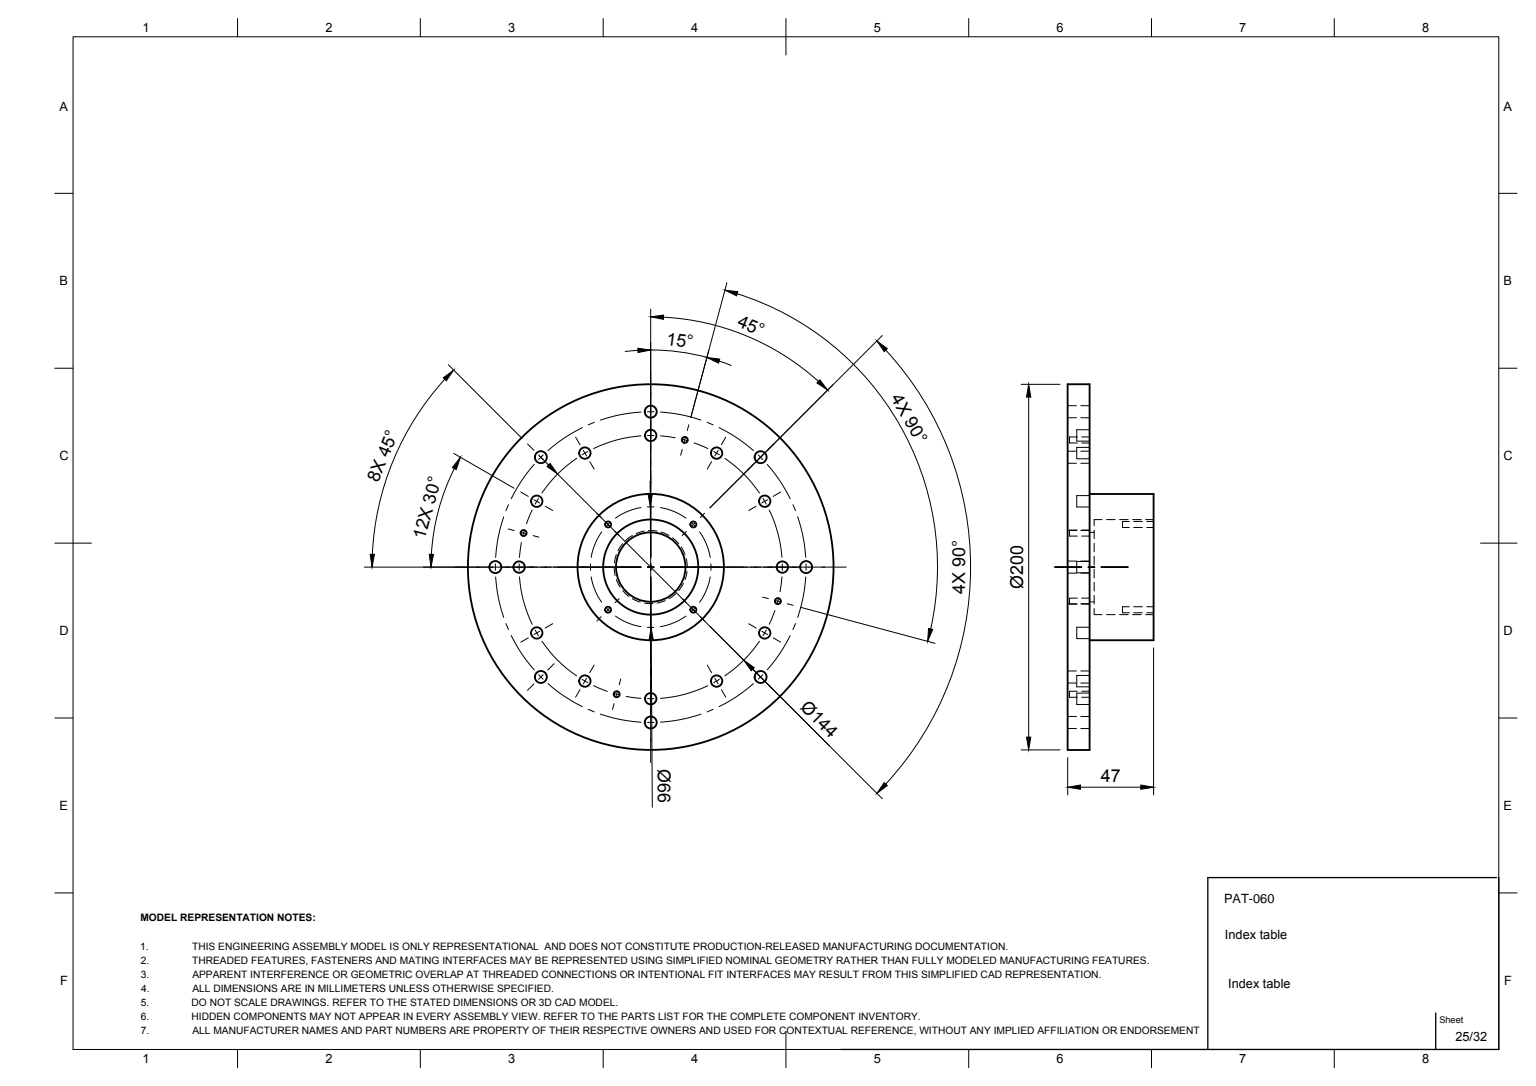
ISO-10303-21;
HEADER;
/* Generated by software containing ST-Developer
 * from STEP Tools, Inc. (www.steptools.com) 
 */

FILE_DESCRIPTION(
/* description */ ('Indexing fixture plate with plunger'),
/* implementation_level */ '2;1');

FILE_NAME(
/* name */ 'Index table.step',
/* time_stamp */ '2026-10-28T03:23:41-07:00',
/* author */ (''),
/* organization */ (''),
/* preprocessor_version */ 'ST-DEVELOPER v20.2',
/* originating_system */ 'Autodesk Translation Framework v15.17.0.0',
/* authorisation */ '');

FILE_SCHEMA (('AUTOMOTIVE_DESIGN { 1 0 10303 214 3 1 1 }'));
ENDSEC;

DATA;
#10=MECHANICAL_DESIGN_GEOMETRIC_PRESENTATION_REPRESENTATION('',(#345),#10020);
#282=SHAPE_REPRESENTATION_RELATIONSHIP('SRR','None',#10158,#309);
#309=ADVANCED_BREP_SHAPE_REPRESENTATION('',(#380),#10011);
#345=STYLED_ITEM('',(#10382),#380);
#380=MANIFOLD_SOLID_BREP('Body1',#4600);
#441=FACE_BOUND('',#1210,.T.);
#442=FACE_BOUND('',#1213,.T.);
#443=FACE_BOUND('',#1215,.T.);
#444=FACE_BOUND('',#1216,.T.);
#445=FACE_BOUND('',#1217,.T.);
#446=FACE_BOUND('',#1218,.T.);
#447=FACE_BOUND('',#1219,.T.);
#448=FACE_BOUND('',#1220,.T.);
#449=FACE_BOUND('',#1221,.T.);
#450=FACE_BOUND('',#1222,.T.);
#451=FACE_BOUND('',#1223,.T.);
#452=FACE_BOUND('',#1224,.T.);
#453=FACE_BOUND('',#1225,.T.);
#454=FACE_BOUND('',#1226,.T.);
#455=FACE_BOUND('',#1227,.T.);
#456=FACE_BOUND('',#1228,.T.);
#457=FACE_BOUND('',#1229,.T.);
#458=FACE_BOUND('',#1230,.T.);
#459=FACE_BOUND('',#1231,.T.);
#460=FACE_BOUND('',#1232,.T.);
#461=FACE_BOUND('',#1233,.T.);
#462=FACE_BOUND('',#1234,.T.);
#463=FACE_BOUND('',#1235,.T.);
#464=FACE_BOUND('',#1236,.T.);
#465=FACE_BOUND('',#1237,.T.);
#466=FACE_BOUND('',#1238,.T.);
#467=FACE_BOUND('',#1239,.T.);
#468=FACE_BOUND('',#1243,.T.);
#469=FACE_BOUND('',#1244,.T.);
#470=FACE_BOUND('',#1245,.T.);
#471=FACE_BOUND('',#1246,.T.);
#472=FACE_BOUND('',#1247,.T.);
#473=FACE_BOUND('',#1248,.T.);
#474=FACE_BOUND('',#1249,.T.);
#475=FACE_BOUND('',#1250,.T.);
#476=FACE_BOUND('',#1251,.T.);
#477=FACE_BOUND('',#1255,.T.);
#478=FACE_BOUND('',#1256,.T.);
#479=FACE_BOUND('',#1257,.T.);
#480=FACE_BOUND('',#1258,.T.);
#481=FACE_BOUND('',#1259,.T.);
#610=PLANE('',#5248);
#611=PLANE('',#5252);
#612=PLANE('',#5256);
#613=PLANE('',#5260);
#614=PLANE('',#5264);
#615=PLANE('',#5268);
#616=PLANE('',#5272);
#617=PLANE('',#5276);
#618=PLANE('',#5280);
#619=PLANE('',#5284);
#620=PLANE('',#5288);
#621=PLANE('',#5292);
#622=PLANE('',#5296);
#623=PLANE('',#5300);
#624=PLANE('',#5304);
#625=PLANE('',#5308);
#626=PLANE('',#5312);
#627=PLANE('',#5316);
#628=PLANE('',#5320);
#629=PLANE('',#5324);
#630=PLANE('',#5349);
#631=PLANE('',#5354);
#632=PLANE('',#5356);
#633=PLANE('',#5363);
#634=PLANE('',#5368);
#821=FACE_OUTER_BOUND('',#1161,.T.);
#822=FACE_OUTER_BOUND('',#1162,.T.);
#823=FACE_OUTER_BOUND('',#1163,.T.);
#824=FACE_OUTER_BOUND('',#1164,.T.);
#825=FACE_OUTER_BOUND('',#1165,.T.);
#826=FACE_OUTER_BOUND('',#1166,.T.);
#827=FACE_OUTER_BOUND('',#1167,.T.);
#828=FACE_OUTER_BOUND('',#1168,.T.);
#829=FACE_OUTER_BOUND('',#1169,.T.);
#830=FACE_OUTER_BOUND('',#1170,.T.);
#831=FACE_OUTER_BOUND('',#1171,.T.);
#832=FACE_OUTER_BOUND('',#1172,.T.);
#833=FACE_OUTER_BOUND('',#1173,.T.);
#834=FACE_OUTER_BOUND('',#1174,.T.);
#835=FACE_OUTER_BOUND('',#1175,.T.);
#836=FACE_OUTER_BOUND('',#1176,.T.);
#837=FACE_OUTER_BOUND('',#1177,.T.);
#838=FACE_OUTER_BOUND('',#1178,.T.);
#839=FACE_OUTER_BOUND('',#1179,.T.);
#840=FACE_OUTER_BOUND('',#1180,.T.);
#841=FACE_OUTER_BOUND('',#1181,.T.);
#842=FACE_OUTER_BOUND('',#1182,.T.);
#843=FACE_OUTER_BOUND('',#1183,.T.);
#844=FACE_OUTER_BOUND('',#1184,.T.);
#845=FACE_OUTER_BOUND('',#1185,.T.);
#846=FACE_OUTER_BOUND('',#1186,.T.);
#847=FACE_OUTER_BOUND('',#1187,.T.);
#848=FACE_OUTER_BOUND('',#1188,.T.);
#849=FACE_OUTER_BOUND('',#1189,.T.);
#850=FACE_OUTER_BOUND('',#1190,.T.);
#851=FACE_OUTER_BOUND('',#1191,.T.);
#852=FACE_OUTER_BOUND('',#1192,.T.);
#853=FACE_OUTER_BOUND('',#1193,.T.);
#854=FACE_OUTER_BOUND('',#1194,.T.);
#855=FACE_OUTER_BOUND('',#1195,.T.);
#856=FACE_OUTER_BOUND('',#1196,.T.);
#857=FACE_OUTER_BOUND('',#1197,.T.);
#858=FACE_OUTER_BOUND('',#1198,.T.);
#859=FACE_OUTER_BOUND('',#1199,.T.);
#860=FACE_OUTER_BOUND('',#1200,.T.);
#861=FACE_OUTER_BOUND('',#1201,.T.);
#862=FACE_OUTER_BOUND('',#1202,.T.);
#863=FACE_OUTER_BOUND('',#1203,.T.);
#864=FACE_OUTER_BOUND('',#1204,.T.);
#865=FACE_OUTER_BOUND('',#1205,.T.);
#866=FACE_OUTER_BOUND('',#1206,.T.);
#867=FACE_OUTER_BOUND('',#1207,.T.);
#868=FACE_OUTER_BOUND('',#1208,.T.);
#869=FACE_OUTER_BOUND('',#1209,.T.);
#870=FACE_OUTER_BOUND('',#1211,.T.);
#871=FACE_OUTER_BOUND('',#1212,.T.);
#872=FACE_OUTER_BOUND('',#1214,.T.);
#873=FACE_OUTER_BOUND('',#1240,.T.);
#874=FACE_OUTER_BOUND('',#1241,.T.);
#875=FACE_OUTER_BOUND('',#1242,.T.);
#876=FACE_OUTER_BOUND('',#1252,.T.);
#877=FACE_OUTER_BOUND('',#1253,.T.);
#878=FACE_OUTER_BOUND('',#1254,.T.);
#1161=EDGE_LOOP('',(#3643,#3644,#3645,#3646));
#1162=EDGE_LOOP('',(#3647));
#1163=EDGE_LOOP('',(#3648,#3649,#3650,#3651));
#1164=EDGE_LOOP('',(#3652));
#1165=EDGE_LOOP('',(#3653,#3654,#3655,#3656));
#1166=EDGE_LOOP('',(#3657));
#1167=EDGE_LOOP('',(#3658,#3659,#3660,#3661));
#1168=EDGE_LOOP('',(#3662));
#1169=EDGE_LOOP('',(#3663,#3664,#3665,#3666));
#1170=EDGE_LOOP('',(#3667));
#1171=EDGE_LOOP('',(#3668,#3669,#3670,#3671));
#1172=EDGE_LOOP('',(#3672));
#1173=EDGE_LOOP('',(#3673,#3674,#3675,#3676));
#1174=EDGE_LOOP('',(#3677));
#1175=EDGE_LOOP('',(#3678,#3679,#3680,#3681));
#1176=EDGE_LOOP('',(#3682));
#1177=EDGE_LOOP('',(#3683,#3684,#3685,#3686));
#1178=EDGE_LOOP('',(#3687));
#1179=EDGE_LOOP('',(#3688,#3689,#3690,#3691));
#1180=EDGE_LOOP('',(#3692));
#1181=EDGE_LOOP('',(#3693,#3694,#3695,#3696));
#1182=EDGE_LOOP('',(#3697));
#1183=EDGE_LOOP('',(#3698,#3699,#3700,#3701));
#1184=EDGE_LOOP('',(#3702));
#1185=EDGE_LOOP('',(#3703,#3704,#3705,#3706));
#1186=EDGE_LOOP('',(#3707));
#1187=EDGE_LOOP('',(#3708,#3709,#3710,#3711));
#1188=EDGE_LOOP('',(#3712));
#1189=EDGE_LOOP('',(#3713,#3714,#3715,#3716));
#1190=EDGE_LOOP('',(#3717));
#1191=EDGE_LOOP('',(#3718,#3719,#3720,#3721));
#1192=EDGE_LOOP('',(#3722));
#1193=EDGE_LOOP('',(#3723,#3724,#3725,#3726));
#1194=EDGE_LOOP('',(#3727));
#1195=EDGE_LOOP('',(#3728,#3729,#3730,#3731));
#1196=EDGE_LOOP('',(#3732));
#1197=EDGE_LOOP('',(#3733,#3734,#3735,#3736));
#1198=EDGE_LOOP('',(#3737));
#1199=EDGE_LOOP('',(#3738,#3739,#3740,#3741));
#1200=EDGE_LOOP('',(#3742));
#1201=EDGE_LOOP('',(#3743,#3744,#3745,#3746));
#1202=EDGE_LOOP('',(#3747,#3748,#3749,#3750));
#1203=EDGE_LOOP('',(#3751,#3752,#3753,#3754));
#1204=EDGE_LOOP('',(#3755,#3756,#3757,#3758));
#1205=EDGE_LOOP('',(#3759,#3760,#3761,#3762));
#1206=EDGE_LOOP('',(#3763,#3764,#3765,#3766));
#1207=EDGE_LOOP('',(#3767,#3768,#3769,#3770));
#1208=EDGE_LOOP('',(#3771,#3772,#3773,#3774));
#1209=EDGE_LOOP('',(#3775));
#1210=EDGE_LOOP('',(#3776));
#1211=EDGE_LOOP('',(#3777,#3778,#3779,#3780));
#1212=EDGE_LOOP('',(#3781));
#1213=EDGE_LOOP('',(#3782));
#1214=EDGE_LOOP('',(#3783));
#1215=EDGE_LOOP('',(#3784));
#1216=EDGE_LOOP('',(#3785));
#1217=EDGE_LOOP('',(#3786));
#1218=EDGE_LOOP('',(#3787));
#1219=EDGE_LOOP('',(#3788));
#1220=EDGE_LOOP('',(#3789));
#1221=EDGE_LOOP('',(#3790));
#1222=EDGE_LOOP('',(#3791));
#1223=EDGE_LOOP('',(#3792));
#1224=EDGE_LOOP('',(#3793));
#1225=EDGE_LOOP('',(#3794));
#1226=EDGE_LOOP('',(#3795));
#1227=EDGE_LOOP('',(#3796));
#1228=EDGE_LOOP('',(#3797));
#1229=EDGE_LOOP('',(#3798));
#1230=EDGE_LOOP('',(#3799));
#1231=EDGE_LOOP('',(#3800));
#1232=EDGE_LOOP('',(#3801));
#1233=EDGE_LOOP('',(#3802));
#1234=EDGE_LOOP('',(#3803));
#1235=EDGE_LOOP('',(#3804));
#1236=EDGE_LOOP('',(#3805));
#1237=EDGE_LOOP('',(#3806));
#1238=EDGE_LOOP('',(#3807));
#1239=EDGE_LOOP('',(#3808));
#1240=EDGE_LOOP('',(#3809,#3810,#3811,#3812));
#1241=EDGE_LOOP('',(#3813,#3814,#3815,#3816));
#1242=EDGE_LOOP('',(#3817));
#1243=EDGE_LOOP('',(#3818));
#1244=EDGE_LOOP('',(#3819));
#1245=EDGE_LOOP('',(#3820));
#1246=EDGE_LOOP('',(#3821));
#1247=EDGE_LOOP('',(#3822));
#1248=EDGE_LOOP('',(#3823));
#1249=EDGE_LOOP('',(#3824));
#1250=EDGE_LOOP('',(#3825));
#1251=EDGE_LOOP('',(#3826));
#1252=EDGE_LOOP('',(#3827,#3828,#3829,#3830));
#1253=EDGE_LOOP('',(#3831,#3832,#3833,#3834));
#1254=EDGE_LOOP('',(#3835));
#1255=EDGE_LOOP('',(#3836));
#1256=EDGE_LOOP('',(#3837));
#1257=EDGE_LOOP('',(#3838));
#1258=EDGE_LOOP('',(#3839));
#1259=EDGE_LOOP('',(#3840));
#1499=LINE('',#9295,#1719);
#1500=LINE('',#9302,#1720);
#1501=LINE('',#9309,#1721);
#1502=LINE('',#9316,#1722);
#1503=LINE('',#9323,#1723);
#1504=LINE('',#9330,#1724);
#1505=LINE('',#9337,#1725);
#1506=LINE('',#9344,#1726);
#1507=LINE('',#9351,#1727);
#1508=LINE('',#9358,#1728);
#1509=LINE('',#9365,#1729);
#1510=LINE('',#9372,#1730);
#1511=LINE('',#9379,#1731);
#1512=LINE('',#9386,#1732);
#1513=LINE('',#9393,#1733);
#1514=LINE('',#9400,#1734);
#1515=LINE('',#9407,#1735);
#1516=LINE('',#9414,#1736);
#1517=LINE('',#9421,#1737);
#1518=LINE('',#9428,#1738);
#1519=LINE('',#9435,#1739);
#1520=LINE('',#9441,#1740);
#1521=LINE('',#9447,#1741);
#1522=LINE('',#9453,#1742);
#1523=LINE('',#9459,#1743);
#1524=LINE('',#9465,#1744);
#1525=LINE('',#9471,#1745);
#1526=LINE('',#9477,#1746);
#1527=LINE('',#9486,#1747);
#1528=LINE('',#9499,#1748);
#1529=LINE('',#9503,#1749);
#1530=LINE('',#9507,#1750);
#1531=LINE('',#9511,#1751);
#1719=VECTOR('',#6360,0.165);
#1720=VECTOR('',#6369,0.165);
#1721=VECTOR('',#6378,0.165);
#1722=VECTOR('',#6387,0.165);
#1723=VECTOR('',#6396,0.31);
#1724=VECTOR('',#6405,0.31);
#1725=VECTOR('',#6414,0.31);
#1726=VECTOR('',#6423,0.31);
#1727=VECTOR('',#6432,0.31);
#1728=VECTOR('',#6441,0.31);
#1729=VECTOR('',#6450,0.31);
#1730=VECTOR('',#6459,0.31);
#1731=VECTOR('',#6468,0.31);
#1732=VECTOR('',#6477,0.31);
#1733=VECTOR('',#6486,0.31);
#1734=VECTOR('',#6495,0.31);
#1735=VECTOR('',#6504,0.165);
#1736=VECTOR('',#6513,0.165);
#1737=VECTOR('',#6522,0.165);
#1738=VECTOR('',#6531,0.165);
#1739=VECTOR('',#6540,0.33);
#1740=VECTOR('',#6547,0.33);
#1741=VECTOR('',#6554,0.33);
#1742=VECTOR('',#6561,0.33);
#1743=VECTOR('',#6568,0.33);
#1744=VECTOR('',#6575,0.33);
#1745=VECTOR('',#6582,0.33);
#1746=VECTOR('',#6589,0.33);
#1747=VECTOR('',#6600,1.9);
#1748=VECTOR('',#6617,2.);
#1749=VECTOR('',#6622,10.);
#1750=VECTOR('',#6627,2.6);
#1751=VECTOR('',#6632,4.);
#1991=CIRCLE('',#5246,0.165);
#1992=CIRCLE('',#5247,0.165);
#1993=CIRCLE('',#5250,0.165);
#1994=CIRCLE('',#5251,0.165);
#1995=CIRCLE('',#5254,0.165);
#1996=CIRCLE('',#5255,0.165);
#1997=CIRCLE('',#5258,0.165);
#1998=CIRCLE('',#5259,0.165);
#1999=CIRCLE('',#5262,0.31);
#2000=CIRCLE('',#5263,0.31);
#2001=CIRCLE('',#5266,0.31);
#2002=CIRCLE('',#5267,0.31);
#2003=CIRCLE('',#5270,0.31);
#2004=CIRCLE('',#5271,0.31);
#2005=CIRCLE('',#5274,0.31);
#2006=CIRCLE('',#5275,0.31);
#2007=CIRCLE('',#5278,0.31);
#2008=CIRCLE('',#5279,0.31);
#2009=CIRCLE('',#5282,0.31);
#2010=CIRCLE('',#5283,0.31);
#2011=CIRCLE('',#5286,0.31);
#2012=CIRCLE('',#5287,0.31);
#2013=CIRCLE('',#5290,0.31);
#2014=CIRCLE('',#5291,0.31);
#2015=CIRCLE('',#5294,0.31);
#2016=CIRCLE('',#5295,0.31);
#2017=CIRCLE('',#5298,0.31);
#2018=CIRCLE('',#5299,0.31);
#2019=CIRCLE('',#5302,0.31);
#2020=CIRCLE('',#5303,0.31);
#2021=CIRCLE('',#5306,0.31);
#2022=CIRCLE('',#5307,0.31);
#2023=CIRCLE('',#5310,0.165);
#2024=CIRCLE('',#5311,0.165);
#2025=CIRCLE('',#5314,0.165);
#2026=CIRCLE('',#5315,0.165);
#2027=CIRCLE('',#5318,0.165);
#2028=CIRCLE('',#5319,0.165);
#2029=CIRCLE('',#5322,0.165);
#2030=CIRCLE('',#5323,0.165);
#2031=CIRCLE('',#5326,0.33);
#2032=CIRCLE('',#5327,0.33);
#2033=CIRCLE('',#5329,0.33);
#2034=CIRCLE('',#5330,0.33);
#2035=CIRCLE('',#5332,0.33);
#2036=CIRCLE('',#5333,0.33);
#2037=CIRCLE('',#5335,0.33);
#2038=CIRCLE('',#5336,0.33);
#2039=CIRCLE('',#5338,0.33);
#2040=CIRCLE('',#5339,0.33);
#2041=CIRCLE('',#5341,0.33);
#2042=CIRCLE('',#5342,0.33);
#2043=CIRCLE('',#5344,0.33);
#2044=CIRCLE('',#5345,0.33);
#2045=CIRCLE('',#5347,0.33);
#2046=CIRCLE('',#5348,0.33);
#2047=CIRCLE('',#5350,2.);
#2048=CIRCLE('',#5351,1.9);
#2049=CIRCLE('',#5353,1.9);
#2050=CIRCLE('',#5355,2.6);
#2051=CIRCLE('',#5357,10.);
#2052=CIRCLE('',#5358,4.);
#2053=CIRCLE('',#5360,2.);
#2054=CIRCLE('',#5362,10.);
#2055=CIRCLE('',#5365,2.6);
#2056=CIRCLE('',#5367,4.);
#2338=VERTEX_POINT('',#9292);
#2339=VERTEX_POINT('',#9294);
#2340=VERTEX_POINT('',#9299);
#2341=VERTEX_POINT('',#9301);
#2342=VERTEX_POINT('',#9306);
#2343=VERTEX_POINT('',#9308);
#2344=VERTEX_POINT('',#9313);
#2345=VERTEX_POINT('',#9315);
#2346=VERTEX_POINT('',#9320);
#2347=VERTEX_POINT('',#9322);
#2348=VERTEX_POINT('',#9327);
#2349=VERTEX_POINT('',#9329);
#2350=VERTEX_POINT('',#9334);
#2351=VERTEX_POINT('',#9336);
#2352=VERTEX_POINT('',#9341);
#2353=VERTEX_POINT('',#9343);
#2354=VERTEX_POINT('',#9348);
#2355=VERTEX_POINT('',#9350);
#2356=VERTEX_POINT('',#9355);
#2357=VERTEX_POINT('',#9357);
#2358=VERTEX_POINT('',#9362);
#2359=VERTEX_POINT('',#9364);
#2360=VERTEX_POINT('',#9369);
#2361=VERTEX_POINT('',#9371);
#2362=VERTEX_POINT('',#9376);
#2363=VERTEX_POINT('',#9378);
#2364=VERTEX_POINT('',#9383);
#2365=VERTEX_POINT('',#9385);
#2366=VERTEX_POINT('',#9390);
#2367=VERTEX_POINT('',#9392);
#2368=VERTEX_POINT('',#9397);
#2369=VERTEX_POINT('',#9399);
#2370=VERTEX_POINT('',#9404);
#2371=VERTEX_POINT('',#9406);
#2372=VERTEX_POINT('',#9411);
#2373=VERTEX_POINT('',#9413);
#2374=VERTEX_POINT('',#9418);
#2375=VERTEX_POINT('',#9420);
#2376=VERTEX_POINT('',#9425);
#2377=VERTEX_POINT('',#9427);
#2378=VERTEX_POINT('',#9432);
#2379=VERTEX_POINT('',#9434);
#2380=VERTEX_POINT('',#9438);
#2381=VERTEX_POINT('',#9440);
#2382=VERTEX_POINT('',#9444);
#2383=VERTEX_POINT('',#9446);
#2384=VERTEX_POINT('',#9450);
#2385=VERTEX_POINT('',#9452);
#2386=VERTEX_POINT('',#9456);
#2387=VERTEX_POINT('',#9458);
#2388=VERTEX_POINT('',#9462);
#2389=VERTEX_POINT('',#9464);
#2390=VERTEX_POINT('',#9468);
#2391=VERTEX_POINT('',#9470);
#2392=VERTEX_POINT('',#9474);
#2393=VERTEX_POINT('',#9476);
#2394=VERTEX_POINT('',#9480);
#2395=VERTEX_POINT('',#9482);
#2396=VERTEX_POINT('',#9485);
#2397=VERTEX_POINT('',#9489);
#2398=VERTEX_POINT('',#9492);
#2399=VERTEX_POINT('',#9494);
#2400=VERTEX_POINT('',#9497);
#2401=VERTEX_POINT('',#9501);
#2402=VERTEX_POINT('',#9506);
#2403=VERTEX_POINT('',#9510);
#2801=EDGE_CURVE('',#2338,#2338,#1991,.T.);
#2802=EDGE_CURVE('',#2338,#2339,#1499,.T.);
#2803=EDGE_CURVE('',#2339,#2339,#1992,.T.);
#2804=EDGE_CURVE('',#2340,#2340,#1993,.T.);
#2805=EDGE_CURVE('',#2340,#2341,#1500,.T.);
#2806=EDGE_CURVE('',#2341,#2341,#1994,.T.);
#2807=EDGE_CURVE('',#2342,#2342,#1995,.T.);
#2808=EDGE_CURVE('',#2342,#2343,#1501,.T.);
#2809=EDGE_CURVE('',#2343,#2343,#1996,.T.);
#2810=EDGE_CURVE('',#2344,#2344,#1997,.T.);
#2811=EDGE_CURVE('',#2344,#2345,#1502,.T.);
#2812=EDGE_CURVE('',#2345,#2345,#1998,.T.);
#2813=EDGE_CURVE('',#2346,#2346,#1999,.T.);
#2814=EDGE_CURVE('',#2346,#2347,#1503,.T.);
#2815=EDGE_CURVE('',#2347,#2347,#2000,.T.);
#2816=EDGE_CURVE('',#2348,#2348,#2001,.T.);
#2817=EDGE_CURVE('',#2348,#2349,#1504,.T.);
#2818=EDGE_CURVE('',#2349,#2349,#2002,.T.);
#2819=EDGE_CURVE('',#2350,#2350,#2003,.T.);
#2820=EDGE_CURVE('',#2350,#2351,#1505,.T.);
#2821=EDGE_CURVE('',#2351,#2351,#2004,.T.);
#2822=EDGE_CURVE('',#2352,#2352,#2005,.T.);
#2823=EDGE_CURVE('',#2352,#2353,#1506,.T.);
#2824=EDGE_CURVE('',#2353,#2353,#2006,.T.);
#2825=EDGE_CURVE('',#2354,#2354,#2007,.T.);
#2826=EDGE_CURVE('',#2354,#2355,#1507,.T.);
#2827=EDGE_CURVE('',#2355,#2355,#2008,.T.);
#2828=EDGE_CURVE('',#2356,#2356,#2009,.T.);
#2829=EDGE_CURVE('',#2356,#2357,#1508,.T.);
#2830=EDGE_CURVE('',#2357,#2357,#2010,.T.);
#2831=EDGE_CURVE('',#2358,#2358,#2011,.T.);
#2832=EDGE_CURVE('',#2358,#2359,#1509,.T.);
#2833=EDGE_CURVE('',#2359,#2359,#2012,.T.);
#2834=EDGE_CURVE('',#2360,#2360,#2013,.T.);
#2835=EDGE_CURVE('',#2360,#2361,#1510,.T.);
#2836=EDGE_CURVE('',#2361,#2361,#2014,.T.);
#2837=EDGE_CURVE('',#2362,#2362,#2015,.T.);
#2838=EDGE_CURVE('',#2362,#2363,#1511,.T.);
#2839=EDGE_CURVE('',#2363,#2363,#2016,.T.);
#2840=EDGE_CURVE('',#2364,#2364,#2017,.T.);
#2841=EDGE_CURVE('',#2364,#2365,#1512,.T.);
#2842=EDGE_CURVE('',#2365,#2365,#2018,.T.);
#2843=EDGE_CURVE('',#2366,#2366,#2019,.T.);
#2844=EDGE_CURVE('',#2366,#2367,#1513,.T.);
#2845=EDGE_CURVE('',#2367,#2367,#2020,.T.);
#2846=EDGE_CURVE('',#2368,#2368,#2021,.T.);
#2847=EDGE_CURVE('',#2368,#2369,#1514,.T.);
#2848=EDGE_CURVE('',#2369,#2369,#2022,.T.);
#2849=EDGE_CURVE('',#2370,#2370,#2023,.T.);
#2850=EDGE_CURVE('',#2370,#2371,#1515,.T.);
#2851=EDGE_CURVE('',#2371,#2371,#2024,.T.);
#2852=EDGE_CURVE('',#2372,#2372,#2025,.T.);
#2853=EDGE_CURVE('',#2372,#2373,#1516,.T.);
#2854=EDGE_CURVE('',#2373,#2373,#2026,.T.);
#2855=EDGE_CURVE('',#2374,#2374,#2027,.T.);
#2856=EDGE_CURVE('',#2374,#2375,#1517,.T.);
#2857=EDGE_CURVE('',#2375,#2375,#2028,.T.);
#2858=EDGE_CURVE('',#2376,#2376,#2029,.T.);
#2859=EDGE_CURVE('',#2376,#2377,#1518,.T.);
#2860=EDGE_CURVE('',#2377,#2377,#2030,.T.);
#2861=EDGE_CURVE('',#2378,#2378,#2031,.T.);
#2862=EDGE_CURVE('',#2378,#2379,#1519,.T.);
#2863=EDGE_CURVE('',#2379,#2379,#2032,.T.);
#2864=EDGE_CURVE('',#2380,#2380,#2033,.T.);
#2865=EDGE_CURVE('',#2380,#2381,#1520,.T.);
#2866=EDGE_CURVE('',#2381,#2381,#2034,.T.);
#2867=EDGE_CURVE('',#2382,#2382,#2035,.T.);
#2868=EDGE_CURVE('',#2382,#2383,#1521,.T.);
#2869=EDGE_CURVE('',#2383,#2383,#2036,.T.);
#2870=EDGE_CURVE('',#2384,#2384,#2037,.T.);
#2871=EDGE_CURVE('',#2384,#2385,#1522,.T.);
#2872=EDGE_CURVE('',#2385,#2385,#2038,.T.);
#2873=EDGE_CURVE('',#2386,#2386,#2039,.T.);
#2874=EDGE_CURVE('',#2386,#2387,#1523,.T.);
#2875=EDGE_CURVE('',#2387,#2387,#2040,.T.);
#2876=EDGE_CURVE('',#2388,#2388,#2041,.T.);
#2877=EDGE_CURVE('',#2388,#2389,#1524,.T.);
#2878=EDGE_CURVE('',#2389,#2389,#2042,.T.);
#2879=EDGE_CURVE('',#2390,#2390,#2043,.T.);
#2880=EDGE_CURVE('',#2390,#2391,#1525,.T.);
#2881=EDGE_CURVE('',#2391,#2391,#2044,.T.);
#2882=EDGE_CURVE('',#2392,#2392,#2045,.T.);
#2883=EDGE_CURVE('',#2392,#2393,#1526,.T.);
#2884=EDGE_CURVE('',#2393,#2393,#2046,.T.);
#2885=EDGE_CURVE('',#2394,#2394,#2047,.T.);
#2886=EDGE_CURVE('',#2395,#2395,#2048,.T.);
#2887=EDGE_CURVE('',#2395,#2396,#1527,.T.);
#2888=EDGE_CURVE('',#2396,#2396,#2049,.T.);
#2889=EDGE_CURVE('',#2397,#2397,#2050,.T.);
#2890=EDGE_CURVE('',#2398,#2398,#2051,.T.);
#2891=EDGE_CURVE('',#2399,#2399,#2052,.T.);
#2892=EDGE_CURVE('',#2400,#2400,#2053,.T.);
#2893=EDGE_CURVE('',#2400,#2394,#1528,.T.);
#2894=EDGE_CURVE('',#2401,#2401,#2054,.T.);
#2895=EDGE_CURVE('',#2401,#2398,#1529,.T.);
#2896=EDGE_CURVE('',#2397,#2402,#1530,.T.);
#2897=EDGE_CURVE('',#2402,#2402,#2055,.T.);
#2898=EDGE_CURVE('',#2399,#2403,#1531,.T.);
#2899=EDGE_CURVE('',#2403,#2403,#2056,.T.);
#3643=ORIENTED_EDGE('',*,*,#2801,.F.);
#3644=ORIENTED_EDGE('',*,*,#2802,.T.);
#3645=ORIENTED_EDGE('',*,*,#2803,.T.);
#3646=ORIENTED_EDGE('',*,*,#2802,.F.);
#3647=ORIENTED_EDGE('',*,*,#2803,.F.);
#3648=ORIENTED_EDGE('',*,*,#2804,.F.);
#3649=ORIENTED_EDGE('',*,*,#2805,.T.);
#3650=ORIENTED_EDGE('',*,*,#2806,.T.);
#3651=ORIENTED_EDGE('',*,*,#2805,.F.);
#3652=ORIENTED_EDGE('',*,*,#2806,.F.);
#3653=ORIENTED_EDGE('',*,*,#2807,.F.);
#3654=ORIENTED_EDGE('',*,*,#2808,.T.);
#3655=ORIENTED_EDGE('',*,*,#2809,.T.);
#3656=ORIENTED_EDGE('',*,*,#2808,.F.);
#3657=ORIENTED_EDGE('',*,*,#2809,.F.);
#3658=ORIENTED_EDGE('',*,*,#2810,.F.);
#3659=ORIENTED_EDGE('',*,*,#2811,.T.);
#3660=ORIENTED_EDGE('',*,*,#2812,.T.);
#3661=ORIENTED_EDGE('',*,*,#2811,.F.);
#3662=ORIENTED_EDGE('',*,*,#2812,.F.);
#3663=ORIENTED_EDGE('',*,*,#2813,.F.);
#3664=ORIENTED_EDGE('',*,*,#2814,.T.);
#3665=ORIENTED_EDGE('',*,*,#2815,.T.);
#3666=ORIENTED_EDGE('',*,*,#2814,.F.);
#3667=ORIENTED_EDGE('',*,*,#2815,.F.);
#3668=ORIENTED_EDGE('',*,*,#2816,.F.);
#3669=ORIENTED_EDGE('',*,*,#2817,.T.);
#3670=ORIENTED_EDGE('',*,*,#2818,.T.);
#3671=ORIENTED_EDGE('',*,*,#2817,.F.);
#3672=ORIENTED_EDGE('',*,*,#2818,.F.);
#3673=ORIENTED_EDGE('',*,*,#2819,.F.);
#3674=ORIENTED_EDGE('',*,*,#2820,.T.);
#3675=ORIENTED_EDGE('',*,*,#2821,.T.);
#3676=ORIENTED_EDGE('',*,*,#2820,.F.);
#3677=ORIENTED_EDGE('',*,*,#2821,.F.);
#3678=ORIENTED_EDGE('',*,*,#2822,.F.);
#3679=ORIENTED_EDGE('',*,*,#2823,.T.);
#3680=ORIENTED_EDGE('',*,*,#2824,.T.);
#3681=ORIENTED_EDGE('',*,*,#2823,.F.);
#3682=ORIENTED_EDGE('',*,*,#2824,.F.);
#3683=ORIENTED_EDGE('',*,*,#2825,.F.);
#3684=ORIENTED_EDGE('',*,*,#2826,.T.);
#3685=ORIENTED_EDGE('',*,*,#2827,.T.);
#3686=ORIENTED_EDGE('',*,*,#2826,.F.);
#3687=ORIENTED_EDGE('',*,*,#2827,.F.);
#3688=ORIENTED_EDGE('',*,*,#2828,.F.);
#3689=ORIENTED_EDGE('',*,*,#2829,.T.);
#3690=ORIENTED_EDGE('',*,*,#2830,.T.);
#3691=ORIENTED_EDGE('',*,*,#2829,.F.);
#3692=ORIENTED_EDGE('',*,*,#2830,.F.);
#3693=ORIENTED_EDGE('',*,*,#2831,.F.);
#3694=ORIENTED_EDGE('',*,*,#2832,.T.);
#3695=ORIENTED_EDGE('',*,*,#2833,.T.);
#3696=ORIENTED_EDGE('',*,*,#2832,.F.);
#3697=ORIENTED_EDGE('',*,*,#2833,.F.);
#3698=ORIENTED_EDGE('',*,*,#2834,.F.);
#3699=ORIENTED_EDGE('',*,*,#2835,.T.);
#3700=ORIENTED_EDGE('',*,*,#2836,.T.);
#3701=ORIENTED_EDGE('',*,*,#2835,.F.);
#3702=ORIENTED_EDGE('',*,*,#2836,.F.);
#3703=ORIENTED_EDGE('',*,*,#2837,.F.);
#3704=ORIENTED_EDGE('',*,*,#2838,.T.);
#3705=ORIENTED_EDGE('',*,*,#2839,.T.);
#3706=ORIENTED_EDGE('',*,*,#2838,.F.);
#3707=ORIENTED_EDGE('',*,*,#2839,.F.);
#3708=ORIENTED_EDGE('',*,*,#2840,.F.);
#3709=ORIENTED_EDGE('',*,*,#2841,.T.);
#3710=ORIENTED_EDGE('',*,*,#2842,.T.);
#3711=ORIENTED_EDGE('',*,*,#2841,.F.);
#3712=ORIENTED_EDGE('',*,*,#2842,.F.);
#3713=ORIENTED_EDGE('',*,*,#2843,.F.);
#3714=ORIENTED_EDGE('',*,*,#2844,.T.);
#3715=ORIENTED_EDGE('',*,*,#2845,.T.);
#3716=ORIENTED_EDGE('',*,*,#2844,.F.);
#3717=ORIENTED_EDGE('',*,*,#2845,.F.);
#3718=ORIENTED_EDGE('',*,*,#2846,.F.);
#3719=ORIENTED_EDGE('',*,*,#2847,.T.);
#3720=ORIENTED_EDGE('',*,*,#2848,.T.);
#3721=ORIENTED_EDGE('',*,*,#2847,.F.);
#3722=ORIENTED_EDGE('',*,*,#2848,.F.);
#3723=ORIENTED_EDGE('',*,*,#2849,.F.);
#3724=ORIENTED_EDGE('',*,*,#2850,.T.);
#3725=ORIENTED_EDGE('',*,*,#2851,.T.);
#3726=ORIENTED_EDGE('',*,*,#2850,.F.);
#3727=ORIENTED_EDGE('',*,*,#2851,.F.);
#3728=ORIENTED_EDGE('',*,*,#2852,.F.);
#3729=ORIENTED_EDGE('',*,*,#2853,.T.);
#3730=ORIENTED_EDGE('',*,*,#2854,.T.);
#3731=ORIENTED_EDGE('',*,*,#2853,.F.);
#3732=ORIENTED_EDGE('',*,*,#2854,.F.);
#3733=ORIENTED_EDGE('',*,*,#2855,.F.);
#3734=ORIENTED_EDGE('',*,*,#2856,.T.);
#3735=ORIENTED_EDGE('',*,*,#2857,.T.);
#3736=ORIENTED_EDGE('',*,*,#2856,.F.);
#3737=ORIENTED_EDGE('',*,*,#2857,.F.);
#3738=ORIENTED_EDGE('',*,*,#2858,.F.);
#3739=ORIENTED_EDGE('',*,*,#2859,.T.);
#3740=ORIENTED_EDGE('',*,*,#2860,.T.);
#3741=ORIENTED_EDGE('',*,*,#2859,.F.);
#3742=ORIENTED_EDGE('',*,*,#2860,.F.);
#3743=ORIENTED_EDGE('',*,*,#2861,.F.);
#3744=ORIENTED_EDGE('',*,*,#2862,.T.);
#3745=ORIENTED_EDGE('',*,*,#2863,.F.);
#3746=ORIENTED_EDGE('',*,*,#2862,.F.);
#3747=ORIENTED_EDGE('',*,*,#2864,.F.);
#3748=ORIENTED_EDGE('',*,*,#2865,.T.);
#3749=ORIENTED_EDGE('',*,*,#2866,.F.);
#3750=ORIENTED_EDGE('',*,*,#2865,.F.);
#3751=ORIENTED_EDGE('',*,*,#2867,.F.);
#3752=ORIENTED_EDGE('',*,*,#2868,.T.);
#3753=ORIENTED_EDGE('',*,*,#2869,.F.);
#3754=ORIENTED_EDGE('',*,*,#2868,.F.);
#3755=ORIENTED_EDGE('',*,*,#2870,.F.);
#3756=ORIENTED_EDGE('',*,*,#2871,.T.);
#3757=ORIENTED_EDGE('',*,*,#2872,.F.);
#3758=ORIENTED_EDGE('',*,*,#2871,.F.);
#3759=ORIENTED_EDGE('',*,*,#2873,.F.);
#3760=ORIENTED_EDGE('',*,*,#2874,.T.);
#3761=ORIENTED_EDGE('',*,*,#2875,.F.);
#3762=ORIENTED_EDGE('',*,*,#2874,.F.);
#3763=ORIENTED_EDGE('',*,*,#2876,.F.);
#3764=ORIENTED_EDGE('',*,*,#2877,.T.);
#3765=ORIENTED_EDGE('',*,*,#2878,.F.);
#3766=ORIENTED_EDGE('',*,*,#2877,.F.);
#3767=ORIENTED_EDGE('',*,*,#2879,.F.);
#3768=ORIENTED_EDGE('',*,*,#2880,.T.);
#3769=ORIENTED_EDGE('',*,*,#2881,.F.);
#3770=ORIENTED_EDGE('',*,*,#2880,.F.);
#3771=ORIENTED_EDGE('',*,*,#2882,.F.);
#3772=ORIENTED_EDGE('',*,*,#2883,.T.);
#3773=ORIENTED_EDGE('',*,*,#2884,.F.);
#3774=ORIENTED_EDGE('',*,*,#2883,.F.);
#3775=ORIENTED_EDGE('',*,*,#2885,.F.);
#3776=ORIENTED_EDGE('',*,*,#2886,.T.);
#3777=ORIENTED_EDGE('',*,*,#2886,.F.);
#3778=ORIENTED_EDGE('',*,*,#2887,.T.);
#3779=ORIENTED_EDGE('',*,*,#2888,.T.);
#3780=ORIENTED_EDGE('',*,*,#2887,.F.);
#3781=ORIENTED_EDGE('',*,*,#2889,.F.);
#3782=ORIENTED_EDGE('',*,*,#2888,.F.);
#3783=ORIENTED_EDGE('',*,*,#2890,.F.);
#3784=ORIENTED_EDGE('',*,*,#2813,.T.);
#3785=ORIENTED_EDGE('',*,*,#2816,.T.);
#3786=ORIENTED_EDGE('',*,*,#2819,.T.);
#3787=ORIENTED_EDGE('',*,*,#2822,.T.);
#3788=ORIENTED_EDGE('',*,*,#2825,.T.);
#3789=ORIENTED_EDGE('',*,*,#2828,.T.);
#3790=ORIENTED_EDGE('',*,*,#2831,.T.);
#3791=ORIENTED_EDGE('',*,*,#2834,.T.);
#3792=ORIENTED_EDGE('',*,*,#2837,.T.);
#3793=ORIENTED_EDGE('',*,*,#2840,.T.);
#3794=ORIENTED_EDGE('',*,*,#2843,.T.);
#3795=ORIENTED_EDGE('',*,*,#2846,.T.);
#3796=ORIENTED_EDGE('',*,*,#2891,.T.);
#3797=ORIENTED_EDGE('',*,*,#2882,.T.);
#3798=ORIENTED_EDGE('',*,*,#2879,.T.);
#3799=ORIENTED_EDGE('',*,*,#2876,.T.);
#3800=ORIENTED_EDGE('',*,*,#2873,.T.);
#3801=ORIENTED_EDGE('',*,*,#2870,.T.);
#3802=ORIENTED_EDGE('',*,*,#2867,.T.);
#3803=ORIENTED_EDGE('',*,*,#2864,.T.);
#3804=ORIENTED_EDGE('',*,*,#2861,.T.);
#3805=ORIENTED_EDGE('',*,*,#2810,.T.);
#3806=ORIENTED_EDGE('',*,*,#2807,.T.);
#3807=ORIENTED_EDGE('',*,*,#2804,.T.);
#3808=ORIENTED_EDGE('',*,*,#2801,.T.);
#3809=ORIENTED_EDGE('',*,*,#2892,.F.);
#3810=ORIENTED_EDGE('',*,*,#2893,.T.);
#3811=ORIENTED_EDGE('',*,*,#2885,.T.);
#3812=ORIENTED_EDGE('',*,*,#2893,.F.);
#3813=ORIENTED_EDGE('',*,*,#2894,.F.);
#3814=ORIENTED_EDGE('',*,*,#2895,.T.);
#3815=ORIENTED_EDGE('',*,*,#2890,.T.);
#3816=ORIENTED_EDGE('',*,*,#2895,.F.);
#3817=ORIENTED_EDGE('',*,*,#2894,.T.);
#3818=ORIENTED_EDGE('',*,*,#2892,.T.);
#3819=ORIENTED_EDGE('',*,*,#2884,.T.);
#3820=ORIENTED_EDGE('',*,*,#2881,.T.);
#3821=ORIENTED_EDGE('',*,*,#2878,.T.);
#3822=ORIENTED_EDGE('',*,*,#2875,.T.);
#3823=ORIENTED_EDGE('',*,*,#2872,.T.);
#3824=ORIENTED_EDGE('',*,*,#2869,.T.);
#3825=ORIENTED_EDGE('',*,*,#2866,.T.);
#3826=ORIENTED_EDGE('',*,*,#2863,.T.);
#3827=ORIENTED_EDGE('',*,*,#2889,.T.);
#3828=ORIENTED_EDGE('',*,*,#2896,.T.);
#3829=ORIENTED_EDGE('',*,*,#2897,.T.);
#3830=ORIENTED_EDGE('',*,*,#2896,.F.);
#3831=ORIENTED_EDGE('',*,*,#2891,.F.);
#3832=ORIENTED_EDGE('',*,*,#2898,.T.);
#3833=ORIENTED_EDGE('',*,*,#2899,.T.);
#3834=ORIENTED_EDGE('',*,*,#2898,.F.);
#3835=ORIENTED_EDGE('',*,*,#2899,.F.);
#3836=ORIENTED_EDGE('',*,*,#2897,.F.);
#3837=ORIENTED_EDGE('',*,*,#2858,.T.);
#3838=ORIENTED_EDGE('',*,*,#2855,.T.);
#3839=ORIENTED_EDGE('',*,*,#2852,.T.);
#3840=ORIENTED_EDGE('',*,*,#2849,.T.);
#4216=CYLINDRICAL_SURFACE('',#5245,0.165);
#4217=CYLINDRICAL_SURFACE('',#5249,0.165);
#4218=CYLINDRICAL_SURFACE('',#5253,0.165);
#4219=CYLINDRICAL_SURFACE('',#5257,0.165);
#4220=CYLINDRICAL_SURFACE('',#5261,0.31);
#4221=CYLINDRICAL_SURFACE('',#5265,0.31);
#4222=CYLINDRICAL_SURFACE('',#5269,0.31);
#4223=CYLINDRICAL_SURFACE('',#5273,0.31);
#4224=CYLINDRICAL_SURFACE('',#5277,0.31);
#4225=CYLINDRICAL_SURFACE('',#5281,0.31);
#4226=CYLINDRICAL_SURFACE('',#5285,0.31);
#4227=CYLINDRICAL_SURFACE('',#5289,0.31);
#4228=CYLINDRICAL_SURFACE('',#5293,0.31);
#4229=CYLINDRICAL_SURFACE('',#5297,0.31);
#4230=CYLINDRICAL_SURFACE('',#5301,0.31);
#4231=CYLINDRICAL_SURFACE('',#5305,0.31);
#4232=CYLINDRICAL_SURFACE('',#5309,0.165);
#4233=CYLINDRICAL_SURFACE('',#5313,0.165);
#4234=CYLINDRICAL_SURFACE('',#5317,0.165);
#4235=CYLINDRICAL_SURFACE('',#5321,0.165);
#4236=CYLINDRICAL_SURFACE('',#5325,0.33);
#4237=CYLINDRICAL_SURFACE('',#5328,0.33);
#4238=CYLINDRICAL_SURFACE('',#5331,0.33);
#4239=CYLINDRICAL_SURFACE('',#5334,0.33);
#4240=CYLINDRICAL_SURFACE('',#5337,0.33);
#4241=CYLINDRICAL_SURFACE('',#5340,0.33);
#4242=CYLINDRICAL_SURFACE('',#5343,0.33);
#4243=CYLINDRICAL_SURFACE('',#5346,0.33);
#4244=CYLINDRICAL_SURFACE('',#5352,1.9);
#4245=CYLINDRICAL_SURFACE('',#5359,2.);
#4246=CYLINDRICAL_SURFACE('',#5361,10.);
#4247=CYLINDRICAL_SURFACE('',#5364,2.6);
#4248=CYLINDRICAL_SURFACE('',#5366,4.);
#4436=ADVANCED_FACE('',(#821),#4216,.F.);
#4437=ADVANCED_FACE('',(#822),#610,.F.);
#4438=ADVANCED_FACE('',(#823),#4217,.F.);
#4439=ADVANCED_FACE('',(#824),#611,.F.);
#4440=ADVANCED_FACE('',(#825),#4218,.F.);
#4441=ADVANCED_FACE('',(#826),#612,.F.);
#4442=ADVANCED_FACE('',(#827),#4219,.F.);
#4443=ADVANCED_FACE('',(#828),#613,.F.);
#4444=ADVANCED_FACE('',(#829),#4220,.F.);
#4445=ADVANCED_FACE('',(#830),#614,.F.);
#4446=ADVANCED_FACE('',(#831),#4221,.F.);
#4447=ADVANCED_FACE('',(#832),#615,.F.);
#4448=ADVANCED_FACE('',(#833),#4222,.F.);
#4449=ADVANCED_FACE('',(#834),#616,.F.);
#4450=ADVANCED_FACE('',(#835),#4223,.F.);
#4451=ADVANCED_FACE('',(#836),#617,.F.);
#4452=ADVANCED_FACE('',(#837),#4224,.F.);
#4453=ADVANCED_FACE('',(#838),#618,.F.);
#4454=ADVANCED_FACE('',(#839),#4225,.F.);
#4455=ADVANCED_FACE('',(#840),#619,.F.);
#4456=ADVANCED_FACE('',(#841),#4226,.F.);
#4457=ADVANCED_FACE('',(#842),#620,.F.);
#4458=ADVANCED_FACE('',(#843),#4227,.F.);
#4459=ADVANCED_FACE('',(#844),#621,.F.);
#4460=ADVANCED_FACE('',(#845),#4228,.F.);
#4461=ADVANCED_FACE('',(#846),#622,.F.);
#4462=ADVANCED_FACE('',(#847),#4229,.F.);
#4463=ADVANCED_FACE('',(#848),#623,.F.);
#4464=ADVANCED_FACE('',(#849),#4230,.F.);
#4465=ADVANCED_FACE('',(#850),#624,.F.);
#4466=ADVANCED_FACE('',(#851),#4231,.F.);
#4467=ADVANCED_FACE('',(#852),#625,.F.);
#4468=ADVANCED_FACE('',(#853),#4232,.F.);
#4469=ADVANCED_FACE('',(#854),#626,.F.);
#4470=ADVANCED_FACE('',(#855),#4233,.F.);
#4471=ADVANCED_FACE('',(#856),#627,.F.);
#4472=ADVANCED_FACE('',(#857),#4234,.F.);
#4473=ADVANCED_FACE('',(#858),#628,.F.);
#4474=ADVANCED_FACE('',(#859),#4235,.F.);
#4475=ADVANCED_FACE('',(#860),#629,.F.);
#4476=ADVANCED_FACE('',(#861),#4236,.F.);
#4477=ADVANCED_FACE('',(#862),#4237,.F.);
#4478=ADVANCED_FACE('',(#863),#4238,.F.);
#4479=ADVANCED_FACE('',(#864),#4239,.F.);
#4480=ADVANCED_FACE('',(#865),#4240,.F.);
#4481=ADVANCED_FACE('',(#866),#4241,.F.);
#4482=ADVANCED_FACE('',(#867),#4242,.F.);
#4483=ADVANCED_FACE('',(#868),#4243,.F.);
#4484=ADVANCED_FACE('',(#869,#441),#630,.T.);
#4485=ADVANCED_FACE('',(#870),#4244,.F.);
#4486=ADVANCED_FACE('',(#871,#442),#631,.F.);
#4487=ADVANCED_FACE('',(#872,#443,#444,#445,#446,#447,#448,#449,#450,#451,
#452,#453,#454,#455,#456,#457,#458,#459,#460,#461,#462,#463,#464,#465,#466,
#467),#632,.F.);
#4488=ADVANCED_FACE('',(#873),#4245,.F.);
#4489=ADVANCED_FACE('',(#874),#4246,.T.);
#4490=ADVANCED_FACE('',(#875,#468,#469,#470,#471,#472,#473,#474,#475,#476),
#633,.T.);
#4491=ADVANCED_FACE('',(#876),#4247,.F.);
#4492=ADVANCED_FACE('',(#877),#4248,.T.);
#4493=ADVANCED_FACE('',(#878,#477,#478,#479,#480,#481),#634,.F.);
#4600=CLOSED_SHELL('',(#4436,#4437,#4438,#4439,#4440,#4441,#4442,#4443,
#4444,#4445,#4446,#4447,#4448,#4449,#4450,#4451,#4452,#4453,#4454,#4455,
#4456,#4457,#4458,#4459,#4460,#4461,#4462,#4463,#4464,#4465,#4466,#4467,
#4468,#4469,#4470,#4471,#4472,#4473,#4474,#4475,#4476,#4477,#4478,#4479,
#4480,#4481,#4482,#4483,#4484,#4485,#4486,#4487,#4488,#4489,#4490,#4491,
#4492,#4493));
#5244=AXIS2_PLACEMENT_3D('',#9290,#6354,#6355);
#5245=AXIS2_PLACEMENT_3D('',#9291,#6356,#6357);
#5246=AXIS2_PLACEMENT_3D('',#9293,#6358,#6359);
#5247=AXIS2_PLACEMENT_3D('',#9296,#6361,#6362);
#5248=AXIS2_PLACEMENT_3D('',#9297,#6363,#6364);
#5249=AXIS2_PLACEMENT_3D('',#9298,#6365,#6366);
#5250=AXIS2_PLACEMENT_3D('',#9300,#6367,#6368);
#5251=AXIS2_PLACEMENT_3D('',#9303,#6370,#6371);
#5252=AXIS2_PLACEMENT_3D('',#9304,#6372,#6373);
#5253=AXIS2_PLACEMENT_3D('',#9305,#6374,#6375);
#5254=AXIS2_PLACEMENT_3D('',#9307,#6376,#6377);
#5255=AXIS2_PLACEMENT_3D('',#9310,#6379,#6380);
#5256=AXIS2_PLACEMENT_3D('',#9311,#6381,#6382);
#5257=AXIS2_PLACEMENT_3D('',#9312,#6383,#6384);
#5258=AXIS2_PLACEMENT_3D('',#9314,#6385,#6386);
#5259=AXIS2_PLACEMENT_3D('',#9317,#6388,#6389);
#5260=AXIS2_PLACEMENT_3D('',#9318,#6390,#6391);
#5261=AXIS2_PLACEMENT_3D('',#9319,#6392,#6393);
#5262=AXIS2_PLACEMENT_3D('',#9321,#6394,#6395);
#5263=AXIS2_PLACEMENT_3D('',#9324,#6397,#6398);
#5264=AXIS2_PLACEMENT_3D('',#9325,#6399,#6400);
#5265=AXIS2_PLACEMENT_3D('',#9326,#6401,#6402);
#5266=AXIS2_PLACEMENT_3D('',#9328,#6403,#6404);
#5267=AXIS2_PLACEMENT_3D('',#9331,#6406,#6407);
#5268=AXIS2_PLACEMENT_3D('',#9332,#6408,#6409);
#5269=AXIS2_PLACEMENT_3D('',#9333,#6410,#6411);
#5270=AXIS2_PLACEMENT_3D('',#9335,#6412,#6413);
#5271=AXIS2_PLACEMENT_3D('',#9338,#6415,#6416);
#5272=AXIS2_PLACEMENT_3D('',#9339,#6417,#6418);
#5273=AXIS2_PLACEMENT_3D('',#9340,#6419,#6420);
#5274=AXIS2_PLACEMENT_3D('',#9342,#6421,#6422);
#5275=AXIS2_PLACEMENT_3D('',#9345,#6424,#6425);
#5276=AXIS2_PLACEMENT_3D('',#9346,#6426,#6427);
#5277=AXIS2_PLACEMENT_3D('',#9347,#6428,#6429);
#5278=AXIS2_PLACEMENT_3D('',#9349,#6430,#6431);
#5279=AXIS2_PLACEMENT_3D('',#9352,#6433,#6434);
#5280=AXIS2_PLACEMENT_3D('',#9353,#6435,#6436);
#5281=AXIS2_PLACEMENT_3D('',#9354,#6437,#6438);
#5282=AXIS2_PLACEMENT_3D('',#9356,#6439,#6440);
#5283=AXIS2_PLACEMENT_3D('',#9359,#6442,#6443);
#5284=AXIS2_PLACEMENT_3D('',#9360,#6444,#6445);
#5285=AXIS2_PLACEMENT_3D('',#9361,#6446,#6447);
#5286=AXIS2_PLACEMENT_3D('',#9363,#6448,#6449);
#5287=AXIS2_PLACEMENT_3D('',#9366,#6451,#6452);
#5288=AXIS2_PLACEMENT_3D('',#9367,#6453,#6454);
#5289=AXIS2_PLACEMENT_3D('',#9368,#6455,#6456);
#5290=AXIS2_PLACEMENT_3D('',#9370,#6457,#6458);
#5291=AXIS2_PLACEMENT_3D('',#9373,#6460,#6461);
#5292=AXIS2_PLACEMENT_3D('',#9374,#6462,#6463);
#5293=AXIS2_PLACEMENT_3D('',#9375,#6464,#6465);
#5294=AXIS2_PLACEMENT_3D('',#9377,#6466,#6467);
#5295=AXIS2_PLACEMENT_3D('',#9380,#6469,#6470);
#5296=AXIS2_PLACEMENT_3D('',#9381,#6471,#6472);
#5297=AXIS2_PLACEMENT_3D('',#9382,#6473,#6474);
#5298=AXIS2_PLACEMENT_3D('',#9384,#6475,#6476);
#5299=AXIS2_PLACEMENT_3D('',#9387,#6478,#6479);
#5300=AXIS2_PLACEMENT_3D('',#9388,#6480,#6481);
#5301=AXIS2_PLACEMENT_3D('',#9389,#6482,#6483);
#5302=AXIS2_PLACEMENT_3D('',#9391,#6484,#6485);
#5303=AXIS2_PLACEMENT_3D('',#9394,#6487,#6488);
#5304=AXIS2_PLACEMENT_3D('',#9395,#6489,#6490);
#5305=AXIS2_PLACEMENT_3D('',#9396,#6491,#6492);
#5306=AXIS2_PLACEMENT_3D('',#9398,#6493,#6494);
#5307=AXIS2_PLACEMENT_3D('',#9401,#6496,#6497);
#5308=AXIS2_PLACEMENT_3D('',#9402,#6498,#6499);
#5309=AXIS2_PLACEMENT_3D('',#9403,#6500,#6501);
#5310=AXIS2_PLACEMENT_3D('',#9405,#6502,#6503);
#5311=AXIS2_PLACEMENT_3D('',#9408,#6505,#6506);
#5312=AXIS2_PLACEMENT_3D('',#9409,#6507,#6508);
#5313=AXIS2_PLACEMENT_3D('',#9410,#6509,#6510);
#5314=AXIS2_PLACEMENT_3D('',#9412,#6511,#6512);
#5315=AXIS2_PLACEMENT_3D('',#9415,#6514,#6515);
#5316=AXIS2_PLACEMENT_3D('',#9416,#6516,#6517);
#5317=AXIS2_PLACEMENT_3D('',#9417,#6518,#6519);
#5318=AXIS2_PLACEMENT_3D('',#9419,#6520,#6521);
#5319=AXIS2_PLACEMENT_3D('',#9422,#6523,#6524);
#5320=AXIS2_PLACEMENT_3D('',#9423,#6525,#6526);
#5321=AXIS2_PLACEMENT_3D('',#9424,#6527,#6528);
#5322=AXIS2_PLACEMENT_3D('',#9426,#6529,#6530);
#5323=AXIS2_PLACEMENT_3D('',#9429,#6532,#6533);
#5324=AXIS2_PLACEMENT_3D('',#9430,#6534,#6535);
#5325=AXIS2_PLACEMENT_3D('',#9431,#6536,#6537);
#5326=AXIS2_PLACEMENT_3D('',#9433,#6538,#6539);
#5327=AXIS2_PLACEMENT_3D('',#9436,#6541,#6542);
#5328=AXIS2_PLACEMENT_3D('',#9437,#6543,#6544);
#5329=AXIS2_PLACEMENT_3D('',#9439,#6545,#6546);
#5330=AXIS2_PLACEMENT_3D('',#9442,#6548,#6549);
#5331=AXIS2_PLACEMENT_3D('',#9443,#6550,#6551);
#5332=AXIS2_PLACEMENT_3D('',#9445,#6552,#6553);
#5333=AXIS2_PLACEMENT_3D('',#9448,#6555,#6556);
#5334=AXIS2_PLACEMENT_3D('',#9449,#6557,#6558);
#5335=AXIS2_PLACEMENT_3D('',#9451,#6559,#6560);
#5336=AXIS2_PLACEMENT_3D('',#9454,#6562,#6563);
#5337=AXIS2_PLACEMENT_3D('',#9455,#6564,#6565);
#5338=AXIS2_PLACEMENT_3D('',#9457,#6566,#6567);
#5339=AXIS2_PLACEMENT_3D('',#9460,#6569,#6570);
#5340=AXIS2_PLACEMENT_3D('',#9461,#6571,#6572);
#5341=AXIS2_PLACEMENT_3D('',#9463,#6573,#6574);
#5342=AXIS2_PLACEMENT_3D('',#9466,#6576,#6577);
#5343=AXIS2_PLACEMENT_3D('',#9467,#6578,#6579);
#5344=AXIS2_PLACEMENT_3D('',#9469,#6580,#6581);
#5345=AXIS2_PLACEMENT_3D('',#9472,#6583,#6584);
#5346=AXIS2_PLACEMENT_3D('',#9473,#6585,#6586);
#5347=AXIS2_PLACEMENT_3D('',#9475,#6587,#6588);
#5348=AXIS2_PLACEMENT_3D('',#9478,#6590,#6591);
#5349=AXIS2_PLACEMENT_3D('',#9479,#6592,#6593);
#5350=AXIS2_PLACEMENT_3D('',#9481,#6594,#6595);
#5351=AXIS2_PLACEMENT_3D('',#9483,#6596,#6597);
#5352=AXIS2_PLACEMENT_3D('',#9484,#6598,#6599);
#5353=AXIS2_PLACEMENT_3D('',#9487,#6601,#6602);
#5354=AXIS2_PLACEMENT_3D('',#9488,#6603,#6604);
#5355=AXIS2_PLACEMENT_3D('',#9490,#6605,#6606);
#5356=AXIS2_PLACEMENT_3D('',#9491,#6607,#6608);
#5357=AXIS2_PLACEMENT_3D('',#9493,#6609,#6610);
#5358=AXIS2_PLACEMENT_3D('',#9495,#6611,#6612);
#5359=AXIS2_PLACEMENT_3D('',#9496,#6613,#6614);
#5360=AXIS2_PLACEMENT_3D('',#9498,#6615,#6616);
#5361=AXIS2_PLACEMENT_3D('',#9500,#6618,#6619);
#5362=AXIS2_PLACEMENT_3D('',#9502,#6620,#6621);
#5363=AXIS2_PLACEMENT_3D('',#9504,#6623,#6624);
#5364=AXIS2_PLACEMENT_3D('',#9505,#6625,#6626);
#5365=AXIS2_PLACEMENT_3D('',#9508,#6628,#6629);
#5366=AXIS2_PLACEMENT_3D('',#9509,#6630,#6631);
#5367=AXIS2_PLACEMENT_3D('',#9512,#6633,#6634);
#5368=AXIS2_PLACEMENT_3D('',#9513,#6635,#6636);
#6354=DIRECTION('axis',(0.,0.,1.));
#6355=DIRECTION('refdir',(1.,0.,0.));
#6356=DIRECTION('center_axis',(0.,0.,1.));
#6357=DIRECTION('ref_axis',(1.,0.,0.));
#6358=DIRECTION('center_axis',(0.,0.,1.));
#6359=DIRECTION('ref_axis',(1.,0.,0.));
#6360=DIRECTION('',(0.,0.,1.));
#6361=DIRECTION('center_axis',(0.,0.,1.));
#6362=DIRECTION('ref_axis',(1.,0.,0.));
#6363=DIRECTION('center_axis',(0.,0.,1.));
#6364=DIRECTION('ref_axis',(1.,0.,0.));
#6365=DIRECTION('center_axis',(0.,0.,1.));
#6366=DIRECTION('ref_axis',(1.,0.,0.));
#6367=DIRECTION('center_axis',(0.,0.,1.));
#6368=DIRECTION('ref_axis',(1.,0.,0.));
#6369=DIRECTION('',(0.,0.,1.));
#6370=DIRECTION('center_axis',(0.,0.,1.));
#6371=DIRECTION('ref_axis',(1.,0.,0.));
#6372=DIRECTION('center_axis',(0.,0.,1.));
#6373=DIRECTION('ref_axis',(1.,0.,0.));
#6374=DIRECTION('center_axis',(0.,0.,1.));
#6375=DIRECTION('ref_axis',(1.,0.,0.));
#6376=DIRECTION('center_axis',(0.,0.,1.));
#6377=DIRECTION('ref_axis',(1.,0.,0.));
#6378=DIRECTION('',(0.,0.,1.));
#6379=DIRECTION('center_axis',(0.,0.,1.));
#6380=DIRECTION('ref_axis',(1.,0.,0.));
#6381=DIRECTION('center_axis',(0.,0.,1.));
#6382=DIRECTION('ref_axis',(1.,0.,0.));
#6383=DIRECTION('center_axis',(0.,0.,1.));
#6384=DIRECTION('ref_axis',(1.,0.,0.));
#6385=DIRECTION('center_axis',(0.,0.,1.));
#6386=DIRECTION('ref_axis',(1.,0.,0.));
#6387=DIRECTION('',(0.,0.,1.));
#6388=DIRECTION('center_axis',(0.,0.,1.));
#6389=DIRECTION('ref_axis',(1.,0.,0.));
#6390=DIRECTION('center_axis',(0.,0.,1.));
#6391=DIRECTION('ref_axis',(1.,0.,0.));
#6392=DIRECTION('center_axis',(0.,0.,1.));
#6393=DIRECTION('ref_axis',(1.,0.,0.));
#6394=DIRECTION('center_axis',(0.,0.,1.));
#6395=DIRECTION('ref_axis',(1.,0.,0.));
#6396=DIRECTION('',(0.,0.,1.));
#6397=DIRECTION('center_axis',(0.,0.,1.));
#6398=DIRECTION('ref_axis',(1.,0.,0.));
#6399=DIRECTION('center_axis',(0.,0.,1.));
#6400=DIRECTION('ref_axis',(1.,0.,0.));
#6401=DIRECTION('center_axis',(0.,0.,1.));
#6402=DIRECTION('ref_axis',(1.,0.,0.));
#6403=DIRECTION('center_axis',(0.,0.,1.));
#6404=DIRECTION('ref_axis',(1.,0.,0.));
#6405=DIRECTION('',(0.,0.,1.));
#6406=DIRECTION('center_axis',(0.,0.,1.));
#6407=DIRECTION('ref_axis',(1.,0.,0.));
#6408=DIRECTION('center_axis',(0.,0.,1.));
#6409=DIRECTION('ref_axis',(1.,0.,0.));
#6410=DIRECTION('center_axis',(0.,0.,1.));
#6411=DIRECTION('ref_axis',(1.,0.,0.));
#6412=DIRECTION('center_axis',(0.,0.,1.));
#6413=DIRECTION('ref_axis',(1.,0.,0.));
#6414=DIRECTION('',(0.,0.,1.));
#6415=DIRECTION('center_axis',(0.,0.,1.));
#6416=DIRECTION('ref_axis',(1.,0.,0.));
#6417=DIRECTION('center_axis',(0.,0.,1.));
#6418=DIRECTION('ref_axis',(1.,0.,0.));
#6419=DIRECTION('center_axis',(0.,0.,1.));
#6420=DIRECTION('ref_axis',(1.,0.,0.));
#6421=DIRECTION('center_axis',(0.,0.,1.));
#6422=DIRECTION('ref_axis',(1.,0.,0.));
#6423=DIRECTION('',(0.,0.,1.));
#6424=DIRECTION('center_axis',(0.,0.,1.));
#6425=DIRECTION('ref_axis',(1.,0.,0.));
#6426=DIRECTION('center_axis',(0.,0.,1.));
#6427=DIRECTION('ref_axis',(1.,0.,0.));
#6428=DIRECTION('center_axis',(0.,0.,1.));
#6429=DIRECTION('ref_axis',(1.,0.,0.));
#6430=DIRECTION('center_axis',(0.,0.,1.));
#6431=DIRECTION('ref_axis',(1.,0.,0.));
#6432=DIRECTION('',(0.,0.,1.));
#6433=DIRECTION('center_axis',(0.,0.,1.));
#6434=DIRECTION('ref_axis',(1.,0.,0.));
#6435=DIRECTION('center_axis',(0.,0.,1.));
#6436=DIRECTION('ref_axis',(1.,0.,0.));
#6437=DIRECTION('center_axis',(0.,0.,1.));
#6438=DIRECTION('ref_axis',(1.,0.,0.));
#6439=DIRECTION('center_axis',(0.,0.,1.));
#6440=DIRECTION('ref_axis',(1.,0.,0.));
#6441=DIRECTION('',(0.,0.,1.));
#6442=DIRECTION('center_axis',(0.,0.,1.));
#6443=DIRECTION('ref_axis',(1.,0.,0.));
#6444=DIRECTION('center_axis',(0.,0.,1.));
#6445=DIRECTION('ref_axis',(1.,0.,0.));
#6446=DIRECTION('center_axis',(0.,0.,1.));
#6447=DIRECTION('ref_axis',(1.,0.,0.));
#6448=DIRECTION('center_axis',(0.,0.,1.));
#6449=DIRECTION('ref_axis',(1.,0.,0.));
#6450=DIRECTION('',(0.,0.,1.));
#6451=DIRECTION('center_axis',(0.,0.,1.));
#6452=DIRECTION('ref_axis',(1.,0.,0.));
#6453=DIRECTION('center_axis',(0.,0.,1.));
#6454=DIRECTION('ref_axis',(1.,0.,0.));
#6455=DIRECTION('center_axis',(0.,0.,1.));
#6456=DIRECTION('ref_axis',(1.,0.,0.));
#6457=DIRECTION('center_axis',(0.,0.,1.));
#6458=DIRECTION('ref_axis',(1.,0.,0.));
#6459=DIRECTION('',(0.,0.,1.));
#6460=DIRECTION('center_axis',(0.,0.,1.));
#6461=DIRECTION('ref_axis',(1.,0.,0.));
#6462=DIRECTION('center_axis',(0.,0.,1.));
#6463=DIRECTION('ref_axis',(1.,0.,0.));
#6464=DIRECTION('center_axis',(0.,0.,1.));
#6465=DIRECTION('ref_axis',(1.,0.,0.));
#6466=DIRECTION('center_axis',(0.,0.,1.));
#6467=DIRECTION('ref_axis',(1.,0.,0.));
#6468=DIRECTION('',(0.,0.,1.));
#6469=DIRECTION('center_axis',(0.,0.,1.));
#6470=DIRECTION('ref_axis',(1.,0.,0.));
#6471=DIRECTION('center_axis',(0.,0.,1.));
#6472=DIRECTION('ref_axis',(1.,0.,0.));
#6473=DIRECTION('center_axis',(0.,0.,1.));
#6474=DIRECTION('ref_axis',(1.,0.,0.));
#6475=DIRECTION('center_axis',(0.,0.,1.));
#6476=DIRECTION('ref_axis',(1.,0.,0.));
#6477=DIRECTION('',(0.,0.,1.));
#6478=DIRECTION('center_axis',(0.,0.,1.));
#6479=DIRECTION('ref_axis',(1.,0.,0.));
#6480=DIRECTION('center_axis',(0.,0.,1.));
#6481=DIRECTION('ref_axis',(1.,0.,0.));
#6482=DIRECTION('center_axis',(0.,0.,1.));
#6483=DIRECTION('ref_axis',(1.,0.,0.));
#6484=DIRECTION('center_axis',(0.,0.,1.));
#6485=DIRECTION('ref_axis',(1.,0.,0.));
#6486=DIRECTION('',(0.,0.,1.));
#6487=DIRECTION('center_axis',(0.,0.,1.));
#6488=DIRECTION('ref_axis',(1.,0.,0.));
#6489=DIRECTION('center_axis',(0.,0.,1.));
#6490=DIRECTION('ref_axis',(1.,0.,0.));
#6491=DIRECTION('center_axis',(0.,0.,1.));
#6492=DIRECTION('ref_axis',(1.,0.,0.));
#6493=DIRECTION('center_axis',(0.,0.,1.));
#6494=DIRECTION('ref_axis',(1.,0.,0.));
#6495=DIRECTION('',(0.,0.,1.));
#6496=DIRECTION('center_axis',(0.,0.,1.));
#6497=DIRECTION('ref_axis',(1.,0.,0.));
#6498=DIRECTION('center_axis',(0.,0.,1.));
#6499=DIRECTION('ref_axis',(1.,0.,0.));
#6500=DIRECTION('center_axis',(0.,0.,1.));
#6501=DIRECTION('ref_axis',(1.,0.,0.));
#6502=DIRECTION('center_axis',(0.,0.,1.));
#6503=DIRECTION('ref_axis',(1.,0.,0.));
#6504=DIRECTION('',(0.,0.,1.));
#6505=DIRECTION('center_axis',(0.,0.,1.));
#6506=DIRECTION('ref_axis',(1.,0.,0.));
#6507=DIRECTION('center_axis',(0.,0.,1.));
#6508=DIRECTION('ref_axis',(1.,0.,0.));
#6509=DIRECTION('center_axis',(0.,0.,1.));
#6510=DIRECTION('ref_axis',(1.,0.,0.));
#6511=DIRECTION('center_axis',(0.,0.,1.));
#6512=DIRECTION('ref_axis',(1.,0.,0.));
#6513=DIRECTION('',(0.,0.,1.));
#6514=DIRECTION('center_axis',(0.,0.,1.));
#6515=DIRECTION('ref_axis',(1.,0.,0.));
#6516=DIRECTION('center_axis',(0.,0.,1.));
#6517=DIRECTION('ref_axis',(1.,0.,0.));
#6518=DIRECTION('center_axis',(0.,0.,1.));
#6519=DIRECTION('ref_axis',(1.,0.,0.));
#6520=DIRECTION('center_axis',(0.,0.,1.));
#6521=DIRECTION('ref_axis',(1.,0.,0.));
#6522=DIRECTION('',(0.,0.,1.));
#6523=DIRECTION('center_axis',(0.,0.,1.));
#6524=DIRECTION('ref_axis',(1.,0.,0.));
#6525=DIRECTION('center_axis',(0.,0.,1.));
#6526=DIRECTION('ref_axis',(1.,0.,0.));
#6527=DIRECTION('center_axis',(0.,0.,1.));
#6528=DIRECTION('ref_axis',(1.,0.,0.));
#6529=DIRECTION('center_axis',(0.,0.,1.));
#6530=DIRECTION('ref_axis',(1.,0.,0.));
#6531=DIRECTION('',(0.,0.,1.));
#6532=DIRECTION('center_axis',(0.,0.,1.));
#6533=DIRECTION('ref_axis',(1.,0.,0.));
#6534=DIRECTION('center_axis',(0.,0.,1.));
#6535=DIRECTION('ref_axis',(1.,0.,0.));
#6536=DIRECTION('center_axis',(0.,0.,1.));
#6537=DIRECTION('ref_axis',(1.,0.,0.));
#6538=DIRECTION('center_axis',(0.,0.,1.));
#6539=DIRECTION('ref_axis',(1.,0.,0.));
#6540=DIRECTION('',(0.,0.,1.));
#6541=DIRECTION('center_axis',(0.,0.,-1.));
#6542=DIRECTION('ref_axis',(1.,0.,0.));
#6543=DIRECTION('center_axis',(0.,0.,1.));
#6544=DIRECTION('ref_axis',(1.,0.,0.));
#6545=DIRECTION('center_axis',(0.,0.,1.));
#6546=DIRECTION('ref_axis',(1.,0.,0.));
#6547=DIRECTION('',(0.,0.,1.));
#6548=DIRECTION('center_axis',(0.,0.,-1.));
#6549=DIRECTION('ref_axis',(1.,0.,0.));
#6550=DIRECTION('center_axis',(0.,0.,1.));
#6551=DIRECTION('ref_axis',(1.,0.,0.));
#6552=DIRECTION('center_axis',(0.,0.,1.));
#6553=DIRECTION('ref_axis',(1.,0.,0.));
#6554=DIRECTION('',(0.,0.,1.));
#6555=DIRECTION('center_axis',(0.,0.,-1.));
#6556=DIRECTION('ref_axis',(1.,0.,0.));
#6557=DIRECTION('center_axis',(0.,0.,1.));
#6558=DIRECTION('ref_axis',(1.,0.,0.));
#6559=DIRECTION('center_axis',(0.,0.,1.));
#6560=DIRECTION('ref_axis',(1.,0.,0.));
#6561=DIRECTION('',(0.,0.,1.));
#6562=DIRECTION('center_axis',(0.,0.,-1.));
#6563=DIRECTION('ref_axis',(1.,0.,0.));
#6564=DIRECTION('center_axis',(0.,0.,1.));
#6565=DIRECTION('ref_axis',(1.,0.,0.));
#6566=DIRECTION('center_axis',(0.,0.,1.));
#6567=DIRECTION('ref_axis',(1.,0.,0.));
#6568=DIRECTION('',(0.,0.,1.));
#6569=DIRECTION('center_axis',(0.,0.,-1.));
#6570=DIRECTION('ref_axis',(1.,0.,0.));
#6571=DIRECTION('center_axis',(0.,0.,1.));
#6572=DIRECTION('ref_axis',(1.,0.,0.));
#6573=DIRECTION('center_axis',(0.,0.,1.));
#6574=DIRECTION('ref_axis',(1.,0.,0.));
#6575=DIRECTION('',(0.,0.,1.));
#6576=DIRECTION('center_axis',(0.,0.,-1.));
#6577=DIRECTION('ref_axis',(1.,0.,0.));
#6578=DIRECTION('center_axis',(0.,0.,1.));
#6579=DIRECTION('ref_axis',(1.,0.,0.));
#6580=DIRECTION('center_axis',(0.,0.,1.));
#6581=DIRECTION('ref_axis',(1.,0.,0.));
#6582=DIRECTION('',(0.,0.,1.));
#6583=DIRECTION('center_axis',(0.,0.,-1.));
#6584=DIRECTION('ref_axis',(1.,0.,0.));
#6585=DIRECTION('center_axis',(0.,0.,1.));
#6586=DIRECTION('ref_axis',(1.,0.,0.));
#6587=DIRECTION('center_axis',(0.,0.,1.));
#6588=DIRECTION('ref_axis',(1.,0.,0.));
#6589=DIRECTION('',(0.,0.,1.));
#6590=DIRECTION('center_axis',(0.,0.,-1.));
#6591=DIRECTION('ref_axis',(1.,0.,0.));
#6592=DIRECTION('center_axis',(0.,0.,1.));
#6593=DIRECTION('ref_axis',(1.,0.,0.));
#6594=DIRECTION('center_axis',(0.,0.,-1.));
#6595=DIRECTION('ref_axis',(1.,0.,0.));
#6596=DIRECTION('center_axis',(0.,0.,-1.));
#6597=DIRECTION('ref_axis',(1.,0.,0.));
#6598=DIRECTION('center_axis',(0.,0.,1.));
#6599=DIRECTION('ref_axis',(1.,0.,0.));
#6600=DIRECTION('',(0.,0.,-1.));
#6601=DIRECTION('center_axis',(0.,0.,-1.));
#6602=DIRECTION('ref_axis',(1.,0.,0.));
#6603=DIRECTION('center_axis',(0.,0.,1.));
#6604=DIRECTION('ref_axis',(1.,0.,0.));
#6605=DIRECTION('center_axis',(0.,0.,1.));
#6606=DIRECTION('ref_axis',(1.,0.,0.));
#6607=DIRECTION('center_axis',(0.,0.,1.));
#6608=DIRECTION('ref_axis',(1.,0.,0.));
#6609=DIRECTION('center_axis',(0.,0.,1.));
#6610=DIRECTION('ref_axis',(1.,0.,0.));
#6611=DIRECTION('center_axis',(0.,0.,1.));
#6612=DIRECTION('ref_axis',(1.,0.,0.));
#6613=DIRECTION('center_axis',(0.,0.,1.));
#6614=DIRECTION('ref_axis',(1.,0.,0.));
#6615=DIRECTION('center_axis',(0.,0.,-1.));
#6616=DIRECTION('ref_axis',(1.,0.,0.));
#6617=DIRECTION('',(0.,0.,-1.));
#6618=DIRECTION('center_axis',(0.,0.,1.));
#6619=DIRECTION('ref_axis',(1.,0.,0.));
#6620=DIRECTION('center_axis',(0.,0.,1.));
#6621=DIRECTION('ref_axis',(1.,0.,0.));
#6622=DIRECTION('',(0.,0.,-1.));
#6623=DIRECTION('center_axis',(0.,0.,1.));
#6624=DIRECTION('ref_axis',(1.,0.,0.));
#6625=DIRECTION('center_axis',(0.,0.,1.));
#6626=DIRECTION('ref_axis',(1.,0.,0.));
#6627=DIRECTION('',(0.,0.,-1.));
#6628=DIRECTION('center_axis',(0.,0.,-1.));
#6629=DIRECTION('ref_axis',(1.,0.,0.));
#6630=DIRECTION('center_axis',(0.,0.,1.));
#6631=DIRECTION('ref_axis',(1.,0.,0.));
#6632=DIRECTION('',(0.,0.,-1.));
#6633=DIRECTION('center_axis',(0.,0.,1.));
#6634=DIRECTION('ref_axis',(1.,0.,0.));
#6635=DIRECTION('center_axis',(0.,0.,1.));
#6636=DIRECTION('ref_axis',(1.,0.,0.));
#9290=CARTESIAN_POINT('',(0.,0.,0.));
#9291=CARTESIAN_POINT('Origin',(-6.95466594928129,-1.86349712473815,6.4));
#9292=CARTESIAN_POINT('',(-7.11966594928129,-1.86349712473815,6.5));
#9293=CARTESIAN_POINT('Origin',(-6.95466594928129,-1.86349712473815,6.5));
#9294=CARTESIAN_POINT('',(-7.11966594928129,-1.86349712473815,7.6));
#9295=CARTESIAN_POINT('',(-7.11966594928129,-1.86349712473815,6.4));
#9296=CARTESIAN_POINT('Origin',(-6.95466594928129,-1.86349712473815,7.6));
#9297=CARTESIAN_POINT('Origin',(-6.95466594928129,-1.86349712473815,7.6));
#9298=CARTESIAN_POINT('Origin',(-1.86349712473815,6.95466594928129,6.4));
#9299=CARTESIAN_POINT('',(-2.02849712473815,6.95466594928129,6.5));
#9300=CARTESIAN_POINT('Origin',(-1.86349712473815,6.95466594928129,6.5));
#9301=CARTESIAN_POINT('',(-2.02849712473815,6.95466594928129,7.6));
#9302=CARTESIAN_POINT('',(-2.02849712473815,6.95466594928129,6.4));
#9303=CARTESIAN_POINT('Origin',(-1.86349712473815,6.95466594928129,7.6));
#9304=CARTESIAN_POINT('Origin',(-1.86349712473815,6.95466594928129,7.6));
#9305=CARTESIAN_POINT('Origin',(6.95466594928129,1.86349712473815,6.4));
#9306=CARTESIAN_POINT('',(6.78966594928129,1.86349712473815,6.5));
#9307=CARTESIAN_POINT('Origin',(6.95466594928129,1.86349712473815,6.5));
#9308=CARTESIAN_POINT('',(6.78966594928129,1.86349712473815,7.6));
#9309=CARTESIAN_POINT('',(6.78966594928129,1.86349712473815,6.4));
#9310=CARTESIAN_POINT('Origin',(6.95466594928129,1.86349712473815,7.6));
#9311=CARTESIAN_POINT('Origin',(6.95466594928129,1.86349712473815,7.6));
#9312=CARTESIAN_POINT('Origin',(1.86349712473815,-6.95466594928129,6.4));
#9313=CARTESIAN_POINT('',(1.69849712473815,-6.95466594928129,6.5));
#9314=CARTESIAN_POINT('Origin',(1.86349712473815,-6.95466594928129,6.5));
#9315=CARTESIAN_POINT('',(1.69849712473815,-6.95466594928129,7.6));
#9316=CARTESIAN_POINT('',(1.69849712473815,-6.95466594928129,6.4));
#9317=CARTESIAN_POINT('Origin',(1.86349712473815,-6.95466594928129,7.6));
#9318=CARTESIAN_POINT('Origin',(1.86349712473815,-6.95466594928129,7.6));
#9319=CARTESIAN_POINT('Origin',(3.6,-6.23538290724796,6.4));
#9320=CARTESIAN_POINT('',(3.29,-6.23538290724796,6.5));
#9321=CARTESIAN_POINT('Origin',(3.6,-6.23538290724796,6.5));
#9322=CARTESIAN_POINT('',(3.29,-6.23538290724796,7.2));
#9323=CARTESIAN_POINT('',(3.29,-6.23538290724796,6.4));
#9324=CARTESIAN_POINT('Origin',(3.6,-6.23538290724796,7.2));
#9325=CARTESIAN_POINT('Origin',(3.6,-6.23538290724796,7.2));
#9326=CARTESIAN_POINT('Origin',(-3.6,-6.23538290724796,6.4));
#9327=CARTESIAN_POINT('',(-3.91,-6.23538290724796,6.5));
#9328=CARTESIAN_POINT('Origin',(-3.6,-6.23538290724796,6.5));
#9329=CARTESIAN_POINT('',(-3.91,-6.23538290724796,7.2));
#9330=CARTESIAN_POINT('',(-3.91,-6.23538290724796,6.4));
#9331=CARTESIAN_POINT('Origin',(-3.6,-6.23538290724796,7.2));
#9332=CARTESIAN_POINT('Origin',(-3.6,-6.23538290724796,7.2));
#9333=CARTESIAN_POINT('Origin',(-7.2,8.81745695386094E-16,6.4));
#9334=CARTESIAN_POINT('',(-7.51,8.43781644612526E-16,6.5));
#9335=CARTESIAN_POINT('Origin',(-7.2,8.81745695386094E-16,6.5));
#9336=CARTESIAN_POINT('',(-7.51,8.43781644612526E-16,7.2));
#9337=CARTESIAN_POINT('',(-7.51,8.43781644612526E-16,6.4));
#9338=CARTESIAN_POINT('Origin',(-7.2,8.81745695386094E-16,7.2));
#9339=CARTESIAN_POINT('Origin',(-7.2,8.88178419700125E-16,7.2));
#9340=CARTESIAN_POINT('Origin',(-6.23538290724796,3.6,6.4));
#9341=CARTESIAN_POINT('',(-6.54538290724796,3.6,6.5));
#9342=CARTESIAN_POINT('Origin',(-6.23538290724796,3.6,6.5));
#9343=CARTESIAN_POINT('',(-6.54538290724796,3.6,7.2));
#9344=CARTESIAN_POINT('',(-6.54538290724796,3.6,6.4));
#9345=CARTESIAN_POINT('Origin',(-6.23538290724796,3.6,7.2));
#9346=CARTESIAN_POINT('Origin',(-6.23538290724796,3.6,7.2));
#9347=CARTESIAN_POINT('Origin',(4.40872847693047E-16,7.2,6.4));
#9348=CARTESIAN_POINT('',(-0.31,7.2,6.5));
#9349=CARTESIAN_POINT('Origin',(4.40872847693047E-16,7.2,6.5));
#9350=CARTESIAN_POINT('',(-0.31,7.2,7.2));
#9351=CARTESIAN_POINT('',(-0.31,7.2,6.4));
#9352=CARTESIAN_POINT('Origin',(4.40872847693047E-16,7.2,7.2));
#9353=CARTESIAN_POINT('Origin',(4.44089209850063E-16,7.2,7.2));
#9354=CARTESIAN_POINT('Origin',(6.23538290724796,3.6,6.4));
#9355=CARTESIAN_POINT('',(5.92538290724796,3.6,6.5));
#9356=CARTESIAN_POINT('Origin',(6.23538290724796,3.6,6.5));
#9357=CARTESIAN_POINT('',(5.92538290724796,3.6,7.2));
#9358=CARTESIAN_POINT('',(5.92538290724796,3.6,6.4));
#9359=CARTESIAN_POINT('Origin',(6.23538290724796,3.6,7.2));
#9360=CARTESIAN_POINT('Origin',(6.23538290724796,3.6,7.2));
#9361=CARTESIAN_POINT('Origin',(3.6,6.23538290724796,6.4));
#9362=CARTESIAN_POINT('',(3.29,6.23538290724796,6.5));
#9363=CARTESIAN_POINT('Origin',(3.6,6.23538290724796,6.5));
#9364=CARTESIAN_POINT('',(3.29,6.23538290724796,7.2));
#9365=CARTESIAN_POINT('',(3.29,6.23538290724796,6.4));
#9366=CARTESIAN_POINT('Origin',(3.6,6.23538290724796,7.2));
#9367=CARTESIAN_POINT('Origin',(3.6,6.23538290724796,7.2));
#9368=CARTESIAN_POINT('Origin',(-3.6,6.23538290724796,6.4));
#9369=CARTESIAN_POINT('',(-3.91,6.23538290724796,6.5));
#9370=CARTESIAN_POINT('Origin',(-3.6,6.23538290724796,6.5));
#9371=CARTESIAN_POINT('',(-3.91,6.23538290724796,7.2));
#9372=CARTESIAN_POINT('',(-3.91,6.23538290724796,6.4));
#9373=CARTESIAN_POINT('Origin',(-3.6,6.23538290724796,7.2));
#9374=CARTESIAN_POINT('Origin',(-3.6,6.23538290724796,7.2));
#9375=CARTESIAN_POINT('Origin',(7.2,0.,6.4));
#9376=CARTESIAN_POINT('',(6.89,-3.79640507735679E-17,6.5));
#9377=CARTESIAN_POINT('Origin',(7.2,0.,6.5));
#9378=CARTESIAN_POINT('',(6.89,-3.79640507735679E-17,7.2));
#9379=CARTESIAN_POINT('',(6.89,-3.79640507735679E-17,6.4));
#9380=CARTESIAN_POINT('Origin',(7.2,0.,7.2));
#9381=CARTESIAN_POINT('Origin',(7.2,0.,7.2));
#9382=CARTESIAN_POINT('Origin',(-6.23538290724796,-3.6,6.4));
#9383=CARTESIAN_POINT('',(-6.54538290724796,-3.6,6.5));
#9384=CARTESIAN_POINT('Origin',(-6.23538290724796,-3.6,6.5));
#9385=CARTESIAN_POINT('',(-6.54538290724796,-3.6,7.2));
#9386=CARTESIAN_POINT('',(-6.54538290724796,-3.6,6.4));
#9387=CARTESIAN_POINT('Origin',(-6.23538290724796,-3.6,7.2));
#9388=CARTESIAN_POINT('Origin',(-6.23538290724796,-3.6,7.2));
#9389=CARTESIAN_POINT('Origin',(-1.32261854307914E-15,-7.2,6.4));
#9390=CARTESIAN_POINT('',(-0.310000000000001,-7.2,6.5));
#9391=CARTESIAN_POINT('Origin',(-1.32261854307914E-15,-7.2,6.5));
#9392=CARTESIAN_POINT('',(-0.310000000000001,-7.2,7.2));
#9393=CARTESIAN_POINT('',(-0.310000000000001,-7.2,6.4));
#9394=CARTESIAN_POINT('Origin',(-1.32261854307914E-15,-7.2,7.2));
#9395=CARTESIAN_POINT('Origin',(-1.33226762955019E-15,-7.2,7.2));
#9396=CARTESIAN_POINT('Origin',(6.23538290724796,-3.6,6.4));
#9397=CARTESIAN_POINT('',(5.92538290724796,-3.6,6.5));
#9398=CARTESIAN_POINT('Origin',(6.23538290724796,-3.6,6.5));
#9399=CARTESIAN_POINT('',(5.92538290724796,-3.6,7.2));
#9400=CARTESIAN_POINT('',(5.92538290724796,-3.6,6.4));
#9401=CARTESIAN_POINT('Origin',(6.23538290724796,-3.6,7.2));
#9402=CARTESIAN_POINT('Origin',(6.23538290724796,-3.6,7.2));
#9403=CARTESIAN_POINT('Origin',(-2.33345237791561,-2.33345237791561,2.9));
#9404=CARTESIAN_POINT('',(-2.49845237791561,-2.33345237791561,3.));
#9405=CARTESIAN_POINT('Origin',(-2.33345237791561,-2.33345237791561,3.));
#9406=CARTESIAN_POINT('',(-2.49845237791561,-2.33345237791561,4.7));
#9407=CARTESIAN_POINT('',(-2.49845237791561,-2.33345237791561,2.9));
#9408=CARTESIAN_POINT('Origin',(-2.33345237791561,-2.33345237791561,4.7));
#9409=CARTESIAN_POINT('Origin',(-2.33345237791561,-2.33345237791561,4.7));
#9410=CARTESIAN_POINT('Origin',(-2.33345237791561,2.33345237791561,2.9));
#9411=CARTESIAN_POINT('',(-2.49845237791561,2.33345237791561,3.));
#9412=CARTESIAN_POINT('Origin',(-2.33345237791561,2.33345237791561,3.));
#9413=CARTESIAN_POINT('',(-2.49845237791561,2.33345237791561,4.7));
#9414=CARTESIAN_POINT('',(-2.49845237791561,2.33345237791561,2.9));
#9415=CARTESIAN_POINT('Origin',(-2.33345237791561,2.33345237791561,4.7));
#9416=CARTESIAN_POINT('Origin',(-2.33345237791561,2.33345237791561,4.7));
#9417=CARTESIAN_POINT('Origin',(2.33345237791561,2.33345237791561,2.9));
#9418=CARTESIAN_POINT('',(2.16845237791561,2.33345237791561,3.));
#9419=CARTESIAN_POINT('Origin',(2.33345237791561,2.33345237791561,3.));
#9420=CARTESIAN_POINT('',(2.16845237791561,2.33345237791561,4.7));
#9421=CARTESIAN_POINT('',(2.16845237791561,2.33345237791561,2.9));
#9422=CARTESIAN_POINT('Origin',(2.33345237791561,2.33345237791561,4.7));
#9423=CARTESIAN_POINT('Origin',(2.33345237791561,2.33345237791561,4.7));
#9424=CARTESIAN_POINT('Origin',(2.33345237791561,-2.33345237791561,2.9));
#9425=CARTESIAN_POINT('',(2.16845237791561,-2.33345237791561,3.));
#9426=CARTESIAN_POINT('Origin',(2.33345237791561,-2.33345237791561,3.));
#9427=CARTESIAN_POINT('',(2.16845237791561,-2.33345237791561,4.7));
#9428=CARTESIAN_POINT('',(2.16845237791561,-2.33345237791561,2.9));
#9429=CARTESIAN_POINT('Origin',(2.33345237791561,-2.33345237791561,4.7));
#9430=CARTESIAN_POINT('Origin',(2.33345237791561,-2.33345237791561,4.7));
#9431=CARTESIAN_POINT('Origin',(-1.56142466891288E-15,-8.5,6.4));
#9432=CARTESIAN_POINT('',(-0.330000000000002,-8.5,6.5));
#9433=CARTESIAN_POINT('Origin',(-1.56142466891288E-15,-8.5,6.5));
#9434=CARTESIAN_POINT('',(-0.330000000000002,-8.5,7.7));
#9435=CARTESIAN_POINT('',(-0.330000000000002,-8.5,6.4));
#9436=CARTESIAN_POINT('Origin',(-1.56142466891288E-15,-8.5,7.7));
#9437=CARTESIAN_POINT('Origin',(-8.5,1.04094977927525E-15,6.4));
#9438=CARTESIAN_POINT('',(-8.83,1.00053643490339E-15,6.5));
#9439=CARTESIAN_POINT('Origin',(-8.5,1.04094977927525E-15,6.5));
#9440=CARTESIAN_POINT('',(-8.83,1.08136312364711E-15,7.7));
#9441=CARTESIAN_POINT('',(-8.83,1.00053643490339E-15,6.4));
#9442=CARTESIAN_POINT('Origin',(-8.5,1.04094977927525E-15,7.7));
#9443=CARTESIAN_POINT('Origin',(-6.01040764008565,6.01040764008565,6.4));
#9444=CARTESIAN_POINT('',(-6.34040764008565,6.01040764008565,6.5));
#9445=CARTESIAN_POINT('Origin',(-6.01040764008565,6.01040764008565,6.5));
#9446=CARTESIAN_POINT('',(-6.34040764008565,6.01040764008565,7.7));
#9447=CARTESIAN_POINT('',(-6.34040764008565,6.01040764008565,6.4));
#9448=CARTESIAN_POINT('Origin',(-6.01040764008565,6.01040764008565,7.7));
#9449=CARTESIAN_POINT('Origin',(6.01040764008565,6.01040764008565,6.4));
#9450=CARTESIAN_POINT('',(5.68040764008565,6.01040764008565,6.5));
#9451=CARTESIAN_POINT('Origin',(6.01040764008565,6.01040764008565,6.5));
#9452=CARTESIAN_POINT('',(5.68040764008565,6.01040764008565,7.7));
#9453=CARTESIAN_POINT('',(5.68040764008565,6.01040764008565,6.4));
#9454=CARTESIAN_POINT('Origin',(6.01040764008565,6.01040764008565,7.7));
#9455=CARTESIAN_POINT('Origin',(5.20474889637625E-16,8.5,6.4));
#9456=CARTESIAN_POINT('',(-0.329999999999999,8.5,6.5));
#9457=CARTESIAN_POINT('Origin',(5.20474889637625E-16,8.5,6.5));
#9458=CARTESIAN_POINT('',(-0.329999999999999,8.5,7.7));
#9459=CARTESIAN_POINT('',(-0.329999999999999,8.5,6.4));
#9460=CARTESIAN_POINT('Origin',(5.20474889637625E-16,8.5,7.7));
#9461=CARTESIAN_POINT('Origin',(8.5,0.,6.4));
#9462=CARTESIAN_POINT('',(8.17,-4.04133443718627E-17,6.5));
#9463=CARTESIAN_POINT('Origin',(8.5,0.,6.5));
#9464=CARTESIAN_POINT('',(8.17,4.04133443718627E-17,7.7));
#9465=CARTESIAN_POINT('',(8.17,-4.04133443718627E-17,6.4));
#9466=CARTESIAN_POINT('Origin',(8.5,0.,7.7));
#9467=CARTESIAN_POINT('Origin',(-6.01040764008566,-6.01040764008565,6.4));
#9468=CARTESIAN_POINT('',(-6.34040764008566,-6.01040764008565,6.5));
#9469=CARTESIAN_POINT('Origin',(-6.01040764008566,-6.01040764008565,6.5));
#9470=CARTESIAN_POINT('',(-6.34040764008566,-6.01040764008565,7.7));
#9471=CARTESIAN_POINT('',(-6.34040764008566,-6.01040764008565,6.4));
#9472=CARTESIAN_POINT('Origin',(-6.01040764008566,-6.01040764008565,7.7));
#9473=CARTESIAN_POINT('Origin',(6.01040764008565,-6.01040764008566,6.4));
#9474=CARTESIAN_POINT('',(5.68040764008565,-6.01040764008566,6.5));
#9475=CARTESIAN_POINT('Origin',(6.01040764008565,-6.01040764008566,6.5));
#9476=CARTESIAN_POINT('',(5.68040764008565,-6.01040764008566,7.7));
#9477=CARTESIAN_POINT('',(5.68040764008565,-6.01040764008566,6.4));
#9478=CARTESIAN_POINT('Origin',(6.01040764008565,-6.01040764008566,7.7));
#9479=CARTESIAN_POINT('Origin',(0.,0.,6.5));
#9480=CARTESIAN_POINT('',(-2.,-2.44929359829471E-16,6.5));
#9481=CARTESIAN_POINT('Origin',(0.,0.,6.5));
#9482=CARTESIAN_POINT('',(-1.9,-2.32682891837997E-16,6.5));
#9483=CARTESIAN_POINT('Origin',(0.,0.,6.5));
#9484=CARTESIAN_POINT('Origin',(0.,0.,6.25));
#9485=CARTESIAN_POINT('',(-1.9,-2.32682891837997E-16,6.25));
#9486=CARTESIAN_POINT('',(-1.9,-2.32682891837997E-16,6.25));
#9487=CARTESIAN_POINT('Origin',(0.,0.,6.25));
#9488=CARTESIAN_POINT('Origin',(0.,0.,6.25));
#9489=CARTESIAN_POINT('',(-2.6,-3.18408167778312E-16,6.25));
#9490=CARTESIAN_POINT('Origin',(0.,0.,6.25));
#9491=CARTESIAN_POINT('Origin',(0.,0.,6.5));
#9492=CARTESIAN_POINT('',(-10.,-1.22464679914735E-15,6.5));
#9493=CARTESIAN_POINT('Origin',(0.,0.,6.5));
#9494=CARTESIAN_POINT('',(-4.,-4.89858719658941E-16,6.5));
#9495=CARTESIAN_POINT('Origin',(0.,0.,6.5));
#9496=CARTESIAN_POINT('Origin',(0.,0.,6.5));
#9497=CARTESIAN_POINT('',(-2.,-2.44929359829471E-16,7.7));
#9498=CARTESIAN_POINT('Origin',(0.,0.,7.7));
#9499=CARTESIAN_POINT('',(-2.,-2.44929359829471E-16,6.5));
#9500=CARTESIAN_POINT('Origin',(0.,0.,6.5));
#9501=CARTESIAN_POINT('',(-10.,-1.22464679914735E-15,7.7));
#9502=CARTESIAN_POINT('Origin',(0.,0.,7.7));
#9503=CARTESIAN_POINT('',(-10.,-1.22464679914735E-15,6.5));
#9504=CARTESIAN_POINT('Origin',(0.,0.,7.7));
#9505=CARTESIAN_POINT('Origin',(0.,0.,3.));
#9506=CARTESIAN_POINT('',(-2.6,-3.18408167778312E-16,3.));
#9507=CARTESIAN_POINT('',(-2.6,-3.18408167778312E-16,3.));
#9508=CARTESIAN_POINT('Origin',(0.,0.,3.));
#9509=CARTESIAN_POINT('Origin',(0.,0.,3.));
#9510=CARTESIAN_POINT('',(-4.,-4.89858719658941E-16,3.));
#9511=CARTESIAN_POINT('',(-4.,-4.89858719658941E-16,3.));
#9512=CARTESIAN_POINT('Origin',(0.,0.,3.));
#9513=CARTESIAN_POINT('Origin',(0.,0.,3.));
#9978=UNCERTAINTY_MEASURE_WITH_UNIT(LENGTH_MEASURE(0.001),#10021,
'DISTANCE_ACCURACY_VALUE',
'Maximum model space distance between geometric entities at asserted c
onnectivities');
#9987=UNCERTAINTY_MEASURE_WITH_UNIT(LENGTH_MEASURE(0.001),#10021,
'DISTANCE_ACCURACY_VALUE',
'Maximum model space distance between geometric entities at asserted c
onnectivities');
#10011=(
GEOMETRIC_REPRESENTATION_CONTEXT(3)
GLOBAL_UNCERTAINTY_ASSIGNED_CONTEXT((#9978))
GLOBAL_UNIT_ASSIGNED_CONTEXT((#10021,#10023,#10024))
REPRESENTATION_CONTEXT('','3D')
);
#10020=(
GEOMETRIC_REPRESENTATION_CONTEXT(3)
GLOBAL_UNCERTAINTY_ASSIGNED_CONTEXT((#9987))
GLOBAL_UNIT_ASSIGNED_CONTEXT((#10021,#10023,#10024))
REPRESENTATION_CONTEXT('','3D')
);
#10021=(
LENGTH_UNIT()
NAMED_UNIT(*)
SI_UNIT(.CENTI.,.METRE.)
);
#10023=(
NAMED_UNIT(*)
PLANE_ANGLE_UNIT()
SI_UNIT($,.RADIAN.)
);
#10024=(
NAMED_UNIT(*)
SI_UNIT($,.STERADIAN.)
SOLID_ANGLE_UNIT()
);
#10048=SHAPE_DEFINITION_REPRESENTATION(#10085,#10158);
#10085=PRODUCT_DEFINITION_SHAPE('',$,#10191);
#10158=SHAPE_REPRESENTATION('',(#5244),#10011);
#10167=PRODUCT_DEFINITION_CONTEXT('part definition',#10265,'design');
#10191=PRODUCT_DEFINITION('Index table','Index table',#10223,#10167);
#10223=PRODUCT_DEFINITION_FORMATION('',$,#10290);
#10265=APPLICATION_CONTEXT(
'Core Data for Automotive Mechanical Design Process');
#10266=PRODUCT_CONTEXT('part definition',#10265,'mechanical');
#10290=PRODUCT('Index table','Index table','Index table',(#10266));
#10376=COLOUR_RGB('Off White',0.89,0.88,0.83);
#10377=FILL_AREA_STYLE_COLOUR('',#10376);
#10378=FILL_AREA_STYLE('',(#10377));
#10379=SURFACE_STYLE_FILL_AREA(#10378);
#10380=SURFACE_SIDE_STYLE('',(#10379));
#10381=SURFACE_STYLE_USAGE(.BOTH.,#10380);
#10382=PRESENTATION_STYLE_ASSIGNMENT((#10381));
ENDSEC;
END-ISO-10303-21;
